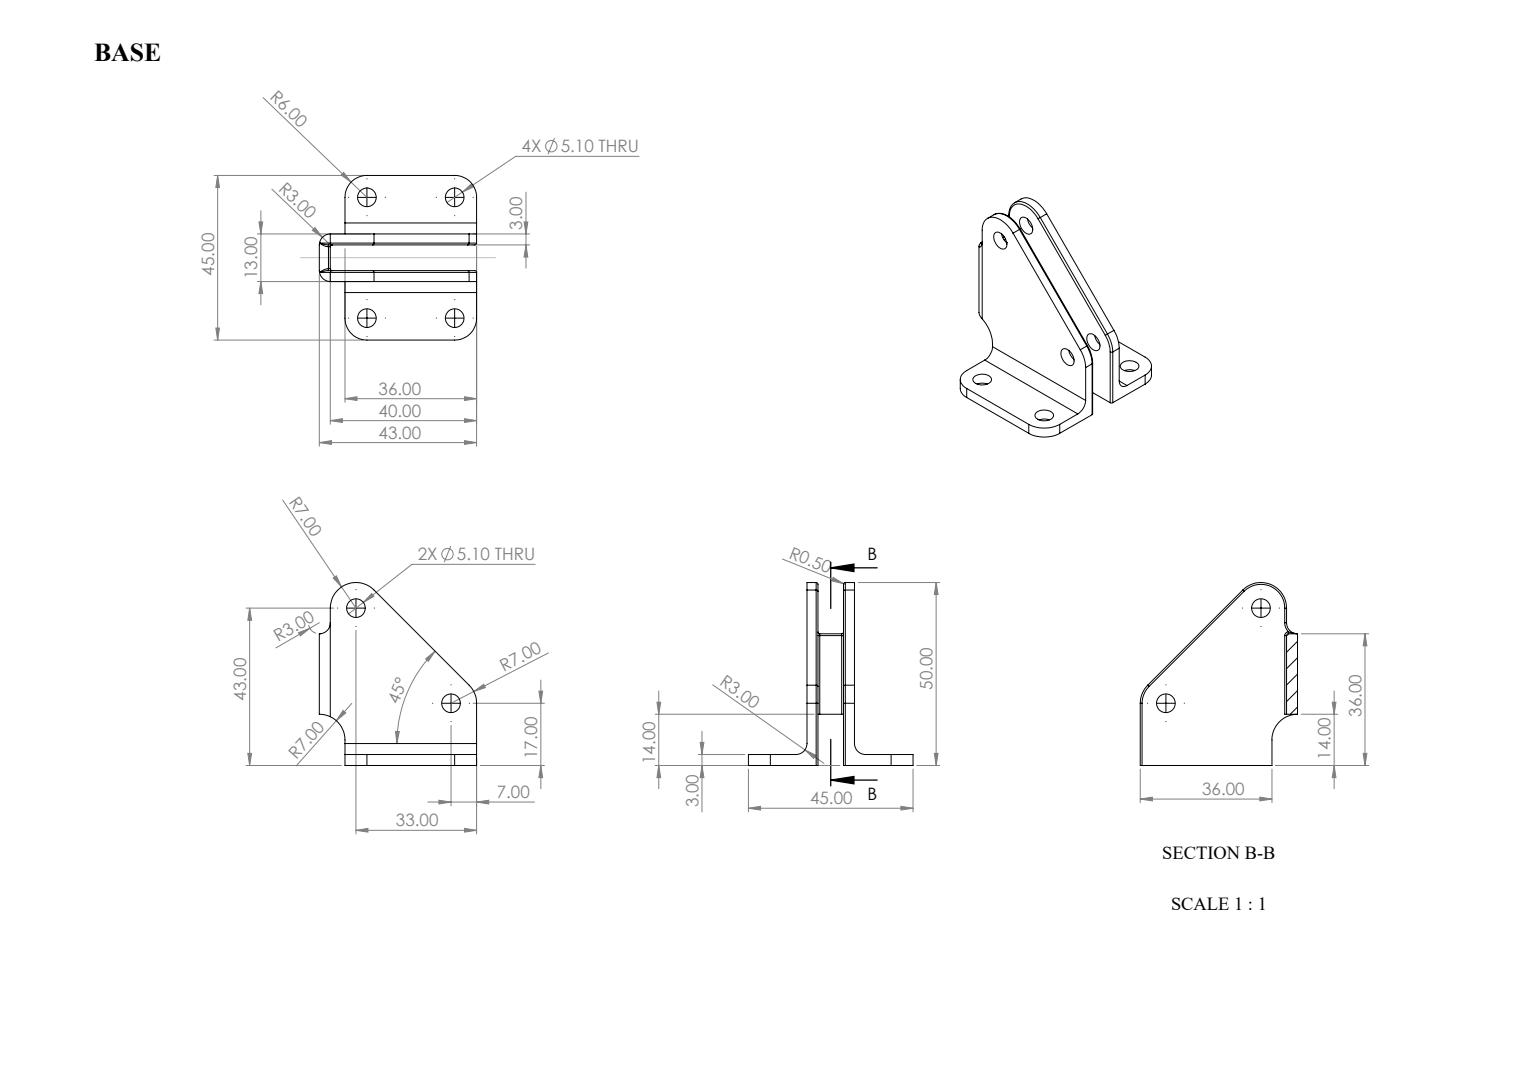
ISO-10303-21;
HEADER;
FILE_DESCRIPTION (('STEP AP214'),
    '1' );
FILE_NAME ('Base.step',
    '2026-10-06T08:09:25',
    ( '' ),
    ( '' ),
    'SwSTEP 2.0',
    'SolidWorks 2021',
    '' );
FILE_SCHEMA (( 'AUTOMOTIVE_DESIGN' ));
ENDSEC;

DATA;
#2=DIRECTION ( 'NONE',  ( -0.000000000000000000, 1.000000000000000000, -0.000000000000000000 ) ) ;
#5=CARTESIAN_POINT ( 'NONE',  ( -4.711587335153455847, 35.99999999900384751, -25.94668155291150313 ) ) ;
#7=AXIS2_PLACEMENT_3D ( 'NONE', #12336, #20843, #10124 ) ;
#19=EDGE_CURVE ( 'NONE', #13411, #2264, #4371, .T. ) ;
#28=ORIENTED_EDGE ( 'NONE', *, *, #13424, .F. ) ;
#32=EDGE_CURVE ( 'NONE', #19371, #4871, #12562, .T. ) ;
#40=CIRCLE ( 'NONE', #19182, 2.550000000000002043 ) ;
#65=ORIENTED_EDGE ( 'NONE', *, *, #2173, .F. ) ;
#84=VERTEX_POINT ( 'NONE', #16838 ) ;
#124=LINE ( 'NONE', #8704, #11013 ) ;
#134=DIRECTION ( 'NONE',  ( 1.000000000000000000, 0.000000000000000000, 0.000000000000000000 ) ) ;
#135=CIRCLE ( 'NONE', #13271, 0.5000000000000004441 ) ;
#145=VERTEX_POINT ( 'NONE', #20516 ) ;
#146=ORIENTED_EDGE ( 'NONE', *, *, #6538, .T. ) ;
#151=AXIS2_PLACEMENT_3D ( 'NONE', #11597, #19127, #20797 ) ;
#166=DIRECTION ( 'NONE',  ( -0.7071067811865475727, -0.7071067811865475727, 0.000000000000000000 ) ) ;
#176=EDGE_LOOP ( 'NONE', ( #1008, #14393, #11718, #4703 ) ) ;
#178=VERTEX_POINT ( 'NONE', #19086 ) ;
#191=STYLED_ITEM ( 'NONE', ( #6397 ), #12837 ) ;
#194=LINE ( 'NONE', #770, #19044 ) ;
#199=ORIENTED_EDGE ( 'NONE', *, *, #4642, .F. ) ;
#204=EDGE_CURVE ( 'NONE', #21236, #14256, #17064, .T. ) ;
#206=FACE_OUTER_BOUND ( 'NONE', #13645, .T. ) ;
#249=VECTOR ( 'NONE', #5863, 1000.000000000000000 ) ;
#250=ORIENTED_EDGE ( 'NONE', *, *, #16395, .F. ) ;
#251=ORIENTED_EDGE ( 'NONE', *, *, #16111, .T. ) ;
#256=DIRECTION ( 'NONE',  ( 0.000000000000000000, -1.000000000000000000, 0.000000000000000000 ) ) ;
#260=CARTESIAN_POINT ( 'NONE',  ( 6.000000000291855429, -0.5000000009961480529, -5.999999999999998224 ) ) ;
#261=DIRECTION ( 'NONE',  ( 0.000000000000000000, 0.000000000000000000, -1.000000000000000000 ) ) ;
#263=LINE ( 'NONE', #5220, #12168 ) ;
#283=VERTEX_POINT ( 'NONE', #1674 ) ;
#297=ADVANCED_FACE ( 'NONE', ( #7100 ), #21448, .T. ) ;
#301=AXIS2_PLACEMENT_3D ( 'NONE', #1691, #21234, #5101 ) ;
#325=EDGE_CURVE ( 'NONE', #4761, #2725, #5554, .T. ) ;
#327=VECTOR ( 'NONE', #12053, 1000.000000000000000 ) ;
#328=CARTESIAN_POINT ( 'NONE',  ( 2.918498775983380256E-10, 2.999999999003851503, -39.00000000000000000 ) ) ;
#334=PLANE ( 'NONE',  #18718 ) ;
#340=CARTESIAN_POINT ( 'NONE',  ( -4.614318463248865854, 37.16513102274245028, -28.94121189041531750 ) ) ;
#343=VERTEX_POINT ( 'NONE', #19786 ) ;
#344=AXIS2_PLACEMENT_3D ( 'NONE', #676, #7844, #18658 ) ;
#348=EDGE_CURVE ( 'NONE', #1547, #16744, #12832, .T. ) ;
#356=CARTESIAN_POINT ( 'NONE',  ( 26.45000000029184051, 16.99999999900385461, -19.00000000000000355 ) ) ;
#371=VERTEX_POINT ( 'NONE', #2699 ) ;
#376=CARTESIAN_POINT ( 'NONE',  ( -3.999999999708139686, 49.99999999900385461, -29.00000000000000355 ) ) ;
#379=DIRECTION ( 'NONE',  ( -0.000000000000000000, -0.000000000000000000, 1.000000000000000000 ) ) ;
#382=CARTESIAN_POINT ( 'NONE',  ( -4.470458892752995794, 37.36863211987452615, -16.03483522404608408 ) ) ;
#383=CYLINDRICAL_SURFACE ( 'NONE', #5439, 2.550000000000000711 ) ;
#412=DIRECTION ( 'NONE',  ( -1.000000000000000000, 0.000000000000000000, 0.000000000000000000 ) ) ;
#414=DIRECTION ( 'NONE',  ( 1.000000000000000000, 0.000000000000000000, 0.000000000000000000 ) ) ;
#459=VECTOR ( 'NONE', #20546, 1000.000000000000000 ) ;
#464=DIRECTION ( 'NONE',  ( 0.000000000000000000, 0.000000000000000000, 1.000000000000000000 ) ) ;
#496=CIRCLE ( 'NONE', #23096, 2.999999999999999112 ) ;
#497=DIRECTION ( 'NONE',  ( -0.7071067811865475727, -0.7071067811865475727, 0.000000000000000000 ) ) ;
#499=DIRECTION ( 'NONE',  ( -1.000000000000000000, -0.000000000000000000, -0.000000000000000000 ) ) ;
#514=AXIS2_PLACEMENT_3D ( 'NONE', #18460, #4209, #9413 ) ;
#516=EDGE_LOOP ( 'NONE', ( #5719, #17219, #15403, #12098, #8144, #13153, #18199, #8414 ) ) ;
#524=EDGE_LOOP ( 'NONE', ( #13786, #13583, #662, #2799 ) ) ;
#536=LINE ( 'NONE', #21829, #14939 ) ;
#548=ORIENTED_EDGE ( 'NONE', *, *, #14303, .F. ) ;
#555=VERTEX_POINT ( 'NONE', #22710 ) ;
#561=CARTESIAN_POINT ( 'NONE',  ( -6.958637496983413051, 36.00028509578874747, -18.50353548315064600 ) ) ;
#569=DIRECTION ( 'NONE',  ( 0.000000000000000000, 0.000000000000000000, 1.000000000000000000 ) ) ;
#603=AXIS2_PLACEMENT_3D ( 'NONE', #12913, #2082, #19970 ) ;
#615=DIRECTION ( 'NONE',  ( 1.000000000000000000, 0.000000000000000000, 0.000000000000000000 ) ) ;
#622=DIRECTION ( 'NONE',  ( -0.7071067811865475727, 0.7071067811865475727, 0.000000000000000000 ) ) ;
#638=CIRCLE ( 'NONE', #21682, 2.550000000000002043 ) ;
#645=AXIS2_PLACEMENT_3D ( 'NONE', #22990, #1692, #8628 ) ;
#662=ORIENTED_EDGE ( 'NONE', *, *, #21476, .T. ) ;
#666=CARTESIAN_POINT ( 'NONE',  ( 2.918498775983380256E-10, 2.999999999003851503, -12.99999999999999822 ) ) ;
#674=AXIS2_PLACEMENT_3D ( 'NONE', #8315, #8440, #20912 ) ;
#676=CARTESIAN_POINT ( 'NONE',  ( 30.00000000029184832, -0.5000000009961480529, -5.999999999999998224 ) ) ;
#688=VERTEX_POINT ( 'NONE', #10911 ) ;
#689=ORIENTED_EDGE ( 'NONE', *, *, #18622, .F. ) ;
#690=VERTEX_POINT ( 'NONE', #12574 ) ;
#692=AXIS2_PLACEMENT_3D ( 'NONE', #16136, #3905, #12614 ) ;
#695=EDGE_LOOP ( 'NONE', ( #13875, #14287, #3852, #8721 ) ) ;
#703=CARTESIAN_POINT ( 'NONE',  ( 36.00000000029184832, 2.999999999003851503, -5.999999999999998224 ) ) ;
#729=CARTESIAN_POINT ( 'NONE',  ( -4.239424077913610311, 37.80035007138371839, -16.00730726111445534 ) ) ;
#731=DIRECTION ( 'NONE',  ( 0.000000000000000000, 0.000000000000000000, 1.000000000000000000 ) ) ;
#736=VECTOR ( 'NONE', #1530, 1000.000000000000000 ) ;
#739=CARTESIAN_POINT ( 'NONE',  ( 6.000000000291855429, -9.961476088449217059E-10, -39.00000000000000000 ) ) ;
#750=LINE ( 'NONE', #7915, #20802 ) ;
#754=DIRECTION ( 'NONE',  ( 0.000000000000000000, 0.000000000000000000, 1.000000000000000000 ) ) ;
#762=DIRECTION ( 'NONE',  ( -0.000000000000000000, 1.000000000000000000, -0.000000000000000000 ) ) ;
#770=CARTESIAN_POINT ( 'NONE',  ( 2.918498775983380256E-10, -9.961476088449217059E-10, -45.00000000000000000 ) ) ;
#775=EDGE_LOOP ( 'NONE', ( #12033, #10591 ) ) ;
#790=CYLINDRICAL_SURFACE ( 'NONE', #17982, 2.550000000000003819 ) ;
#818=DIRECTION ( 'NONE',  ( -0.000000000000000000, 1.000000000000000000, -0.000000000000000000 ) ) ;
#819=CARTESIAN_POINT ( 'NONE',  ( 2.918498775983380256E-10, 2.999999999003851503, -29.00000000000000355 ) ) ;
#820=LINE ( 'NONE', #15157, #19828 ) ;
#827=ORIENTED_EDGE ( 'NONE', *, *, #22142, .T. ) ;
#832=DIRECTION ( 'NONE',  ( -1.000000000000000000, 0.000000000000000000, 0.000000000000000000 ) ) ;
#839=DIRECTION ( 'NONE',  ( 0.7071067811865474617, -0.7071067811865474617, 0.000000000000000000 ) ) ;
#845=DIRECTION ( 'NONE',  ( 0.000000000000000000, 1.000000000000000000, 0.000000000000000000 ) ) ;
#856=AXIS2_PLACEMENT_3D ( 'NONE', #18442, #7510, #21754 ) ;
#866=EDGE_LOOP ( 'NONE', ( #15194, #20184, #2377, #21781 ) ) ;
#888=VERTEX_POINT ( 'NONE', #16668 ) ;
#889=VECTOR ( 'NONE', #18743, 1000.000000000000000 ) ;
#944=DIRECTION ( 'NONE',  ( -1.000000000000000000, -0.000000000000000000, -0.000000000000000000 ) ) ;
#946=CARTESIAN_POINT ( 'NONE',  ( -6.999999999708142795, 38.99999999900385461, -19.00000000000000355 ) ) ;
#949=ORIENTED_EDGE ( 'NONE', *, *, #8818, .F. ) ;
#974=EDGE_CURVE ( 'NONE', #18076, #3151, #3624, .T. ) ;
#983=EDGE_LOOP ( 'NONE', ( #1133, #3126, #6569, #4982 ) ) ;
#984=CARTESIAN_POINT ( 'NONE',  ( -6.999999999708142795, 13.99999999900385106, -22.50000000000000000 ) ) ;
#987=FACE_OUTER_BOUND ( 'NONE', #17816, .T. ) ;
#989=DIRECTION ( 'NONE',  ( -0.000000000000000000, -0.000000000000000000, 1.000000000000000000 ) ) ;
#993=CARTESIAN_POINT ( 'NONE',  ( 30.00000000029184832, -9.961476088449217059E-10, -39.00000000000000000 ) ) ;
#996=FACE_OUTER_BOUND ( 'NONE', #14966, .T. ) ;
#1008=ORIENTED_EDGE ( 'NONE', *, *, #19202, .T. ) ;
#1009=ORIENTED_EDGE ( 'NONE', *, *, #10614, .F. ) ;
#1010=AXIS2_PLACEMENT_3D ( 'NONE', #8199, #4301, #10078 ) ;
#1013=VECTOR ( 'NONE', #7217, 1000.000000000000000 ) ;
#1016=DIRECTION ( 'NONE',  ( 1.000000000000000000, -1.858632295689435609E-16, 0.000000000000000000 ) ) ;
#1017=DIRECTION ( 'NONE',  ( 1.000000000000000000, 0.000000000000000000, 0.000000000000000000 ) ) ;
#1018=ADVANCED_FACE ( 'NONE', ( #13625 ), #18923, .F. ) ;
#1020=CARTESIAN_POINT ( 'NONE',  ( -6.999999999708142795, 35.99999999900384751, -22.50000000000000000 ) ) ;
#1024=FACE_BOUND ( 'NONE', #9944, .T. ) ;
#1027=B_SPLINE_CURVE_WITH_KNOTS ( 'NONE', 3,
 ( #21795, #5679, #12838, #11417, #18604, #18254, #22246, #4347, #6134, #2477, #9315, #9656, #13313, #16811, #382, #729, #20493, #11527, #16358, #21901 ),
 .UNSPECIFIED., .F., .F.,
 ( 4, 2, 2, 2, 2, 2, 2, 2, 2, 4 ),
 ( 0.0005000078514897923158, 0.001232179299099195411, 0.001964350746708598289, 0.002696522194318001601, 0.003062607918122696102, 0.003428693641927389735, 0.004160865089536783072, 0.004893036537146174675, 0.005625207984755568012, 0.006357379432364960482 ),
 .UNSPECIFIED. ) ;
#1034=FACE_OUTER_BOUND ( 'NONE', #5261, .T. ) ;
#1036=AXIS2_PLACEMENT_3D ( 'NONE', #946, #10108, #20935 ) ;
#1046=FACE_OUTER_BOUND ( 'NONE', #14257, .T. ) ;
#1058=EDGE_CURVE ( 'NONE', #11848, #1430, #638, .T. ) ;
#1061=DIRECTION ( 'NONE',  ( -1.613696256722611405E-16, 0.000000000000000000, -1.000000000000000000 ) ) ;
#1066=AXIS2_PLACEMENT_3D ( 'NONE', #3230, #21463, #8745 ) ;
#1068=ADVANCED_FACE ( 'NONE', ( #1046 ), #15491, .F. ) ;
#1077=CARTESIAN_POINT ( 'NONE',  ( -6.549842551586334771, 36.00336057837468928, -26.38138186026117893 ) ) ;
#1082=CARTESIAN_POINT ( 'NONE',  ( 35.50000000029184832, 2.999999999003851503, -19.00000000000000355 ) ) ;
#1087=CARTESIAN_POINT ( 'NONE',  ( 35.50000000029184832, 2.999999999003851503, -18.50000000000000355 ) ) ;
#1090=AXIS2_PLACEMENT_3D ( 'NONE', #17003, #17354, #15598 ) ;
#1103=ORIENTED_EDGE ( 'NONE', *, *, #6153, .T. ) ;
#1127=ORIENTED_EDGE ( 'NONE', *, *, #8585, .T. ) ;
#1130=AXIS2_PLACEMENT_3D ( 'NONE', #16695, #21064, #22587 ) ;
#1133=ORIENTED_EDGE ( 'NONE', *, *, #7575, .T. ) ;
#1137=DIRECTION ( 'NONE',  ( 0.000000000000000000, -1.000000000000000000, 0.000000000000000000 ) ) ;
#1142=CARTESIAN_POINT ( 'NONE',  ( -6.962001439796708269, 35.99999999900384751, -26.47597002942762145 ) ) ;
#1153=EDGE_CURVE ( 'NONE', #19243, #10116, #19375, .T. ) ;
#1163=DIRECTION ( 'NONE',  ( 0.000000000000000000, 0.000000000000000000, 1.000000000000000000 ) ) ;
#1169=CARTESIAN_POINT ( 'NONE',  ( 2.918498775983380256E-10, 6.999999999003851947, -26.00000000000000000 ) ) ;
#1181=ORIENTED_EDGE ( 'NONE', *, *, #21353, .T. ) ;
#1234=ORIENTED_EDGE ( 'NONE', *, *, #8668, .F. ) ;
#1245=ORIENTED_EDGE ( 'NONE', *, *, #3629, .T. ) ;
#1257=VECTOR ( 'NONE', #20720, 1000.000000000000000 ) ;
#1267=ORIENTED_EDGE ( 'NONE', *, *, #2745, .T. ) ;
#1276=AXIS2_PLACEMENT_3D ( 'NONE', #16097, #15759, #12105 ) ;
#1296=TOROIDAL_SURFACE ( 'NONE', #11415, 6.500000000000000888, 0.5000000000000000000 ) ;
#1305=ORIENTED_EDGE ( 'NONE', *, *, #10538, .T. ) ;
#1325=VECTOR ( 'NONE', #1887, 1000.000000000000000 ) ;
#1354=ORIENTED_EDGE ( 'NONE', *, *, #16873, .F. ) ;
#1364=DIRECTION ( 'NONE',  ( 1.000000000000000000, 0.000000000000000000, 0.000000000000000000 ) ) ;
#1370=CARTESIAN_POINT ( 'NONE',  ( -6.959227686631209941, 36.00023952070644384, -18.50706566189541391 ) ) ;
#1376=CARTESIAN_POINT ( 'NONE',  ( -5.786576545576803454, 13.89610628501159795, -16.58192921595065883 ) ) ;
#1412=AXIS2_PLACEMENT_3D ( 'NONE', #8513, #19100, #13917 ) ;
#1413=ORIENTED_EDGE ( 'NONE', *, *, #10933, .T. ) ;
#1425=APPLICATION_CONTEXT ( 'automotive_design' ) ;
#1430=VERTEX_POINT ( 'NONE', #15434 ) ;
#1432=ADVANCED_FACE ( 'NONE', ( #22976 ), #12015, .F. ) ;
#1451=DIRECTION ( 'NONE',  ( 0.000000000000000000, 1.000000000000000000, -0.000000000000000000 ) ) ;
#1500=CARTESIAN_POINT ( 'NONE',  ( 29.00000000029184832, 16.99999999900385461, -25.50000000000000355 ) ) ;
#1510=DIRECTION ( 'NONE',  ( 1.000000000000000000, -0.000000000000000000, -0.000000000000000000 ) ) ;
#1520=VERTEX_POINT ( 'NONE', #10375 ) ;
#1530=DIRECTION ( 'NONE',  ( -1.000000000000000000, 0.000000000000000000, -0.000000000000000000 ) ) ;
#1534=DIRECTION ( 'NONE',  ( -1.000000000000000000, 0.000000000000000000, 0.000000000000000000 ) ) ;
#1537=AXIS2_PLACEMENT_3D ( 'NONE', #19881, #3750, #9051 ) ;
#1541=EDGE_LOOP ( 'NONE', ( #19704, #15907, #14735, #4989 ) ) ;
#1544=ORIENTED_EDGE ( 'NONE', *, *, #20662, .F. ) ;
#1547=VERTEX_POINT ( 'NONE', #5448 ) ;
#1577=CARTESIAN_POINT ( 'NONE',  ( 2.918498775983380256E-10, -9.961476088449217059E-10, -26.00000000000000000 ) ) ;
#1597=EDGE_CURVE ( 'NONE', #20279, #8964, #13375, .T. ) ;
#1602=ORIENTED_EDGE ( 'NONE', *, *, #4180, .F. ) ;
#1628=EDGE_CURVE ( 'NONE', #14201, #16629, #12993, .T. ) ;
#1648=EDGE_CURVE ( 'NONE', #15365, #9160, #13753, .T. ) ;
#1655=VECTOR ( 'NONE', #17115, 1000.000000000000000 ) ;
#1665=VERTEX_POINT ( 'NONE', #15051 ) ;
#1670=AXIS2_PLACEMENT_3D ( 'NONE', #6502, #15199, #22268 ) ;
#1674=CARTESIAN_POINT ( 'NONE',  ( -3.999999999708153453, 38.99999999900385461, -15.99999999999999289 ) ) ;
#1681=EDGE_CURVE ( 'NONE', #8658, #12443, #16806, .T. ) ;
#1683=FACE_OUTER_BOUND ( 'NONE', #1741, .T. ) ;
#1688=LINE ( 'NONE', #5330, #1013 ) ;
#1691=CARTESIAN_POINT ( 'NONE',  ( -4.499999999708154341, 35.49999999900384751, -25.50000000000000000 ) ) ;
#1692=DIRECTION ( 'NONE',  ( 0.000000000000000000, 0.000000000000000000, 1.000000000000000000 ) ) ;
#1703=DIRECTION ( 'NONE',  ( -1.858632295689435609E-16, -1.000000000000000000, 0.000000000000000000 ) ) ;
#1710=PLANE ( 'NONE',  #19487 ) ;
#1720=ORIENTED_EDGE ( 'NONE', *, *, #15193, .T. ) ;
#1722=ORIENTED_EDGE ( 'NONE', *, *, #14532, .T. ) ;
#1741=EDGE_LOOP ( 'NONE', ( #12035, #6194, #22439, #10055 ) ) ;
#1747=AXIS2_PLACEMENT_3D ( 'NONE', #8327, #15376, #7978 ) ;
#1765=CARTESIAN_POINT ( 'NONE',  ( -4.499999999708154341, 35.99999999900384751, -22.50000000000000000 ) ) ;
#1780=CARTESIAN_POINT ( 'NONE',  ( -6.962001439796708269, 35.99999999900384751, -26.47597002942762145 ) ) ;
#1782=CARTESIAN_POINT ( 'NONE',  ( 29.00000000029184832, 16.99999999900385461, -18.50000000000000355 ) ) ;
#1787=EDGE_CURVE ( 'NONE', #9785, #9160, #6352, .T. ) ;
#1802=ORIENTED_EDGE ( 'NONE', *, *, #17536, .F. ) ;
#1811=ORIENTED_EDGE ( 'NONE', *, *, #2933, .F. ) ;
#1820=DIRECTION ( 'NONE',  ( 0.000000000000000000, 0.000000000000000000, 1.000000000000000000 ) ) ;
#1824=CARTESIAN_POINT ( 'NONE',  ( -4.365918574175959854, 13.48846683486500808, -16.01652206364978781 ) ) ;
#1833=ORIENTED_EDGE ( 'NONE', *, *, #348, .F. ) ;
#1834=VERTEX_POINT ( 'NONE', #19062 ) ;
#1842=DIRECTION ( 'NONE',  ( 0.000000000000000000, -0.000000000000000000, -1.000000000000000000 ) ) ;
#1845=LINE ( 'NONE', #5152, #3945 ) ;
#1857=ORIENTED_EDGE ( 'NONE', *, *, #6505, .F. ) ;
#1858=CARTESIAN_POINT ( 'NONE',  ( -6.226186441994419063, 36.09747688189035131, -28.02588720118439269 ) ) ;
#1887=DIRECTION ( 'NONE',  ( 0.000000000000000000, -1.000000000000000000, 0.000000000000000000 ) ) ;
#1891=CARTESIAN_POINT ( 'NONE',  ( 0.4500000002918510544, 42.99999999900385461, -15.99999999999999289 ) ) ;
#1911=ORIENTED_EDGE ( 'NONE', *, *, #17784, .T. ) ;
#1914=ORIENTED_EDGE ( 'NONE', *, *, #5831, .T. ) ;
#1915=ORIENTED_EDGE ( 'NONE', *, *, #4798, .F. ) ;
#1916=EDGE_LOOP ( 'NONE', ( #16349, #12628 ) ) ;
#1933=CARTESIAN_POINT ( 'NONE',  ( 5.550000000291854363, 42.99999999900385461, -25.50000000000000355 ) ) ;
#1952=FACE_BOUND ( 'NONE', #15450, .T. ) ;
#1954=CARTESIAN_POINT ( 'NONE',  ( 2.918498775983380256E-10, -9.961476088449217059E-10, -19.00000000000000355 ) ) ;
#1974=CARTESIAN_POINT ( 'NONE',  ( -6.959810536856695151, 36.00015702695179698, -18.51059057611807646 ) ) ;
#1993=CIRCLE ( 'NONE', #20796, 0.5000000000000004441 ) ;
#2011=CIRCLE ( 'NONE', #9164, 2.550000000000002043 ) ;
#2025=CARTESIAN_POINT ( 'NONE',  ( -5.416517661024267127, 35.99999999900385461, -19.34908248715211698 ) ) ;
#2035=ORIENTED_EDGE ( 'NONE', *, *, #21054, .T. ) ;
#2041=ORIENTED_EDGE ( 'NONE', *, *, #13149, .F. ) ;
#2049=LINE ( 'NONE', #18181, #15713 ) ;
#2054=FACE_OUTER_BOUND ( 'NONE', #6213, .T. ) ;
#2057=CYLINDRICAL_SURFACE ( 'NONE', #5233, 3.000000000000002665 ) ;
#2058=ORIENTED_EDGE ( 'NONE', *, *, #21821, .T. ) ;
#2068=DIRECTION ( 'NONE',  ( -0.000000000000000000, -0.000000000000000000, 1.000000000000000000 ) ) ;
#2075=CARTESIAN_POINT ( 'NONE',  ( 6.000000000291855429, -9.961476088449217059E-10, -5.999999999999998224 ) ) ;
#2076=DIRECTION ( 'NONE',  ( 0.000000000000000000, 0.000000000000000000, -1.000000000000000000 ) ) ;
#2079=CARTESIAN_POINT ( 'NONE',  ( -3.999999999708153453, 13.99999999900385106, -25.50000000000000000 ) ) ;
#2082=DIRECTION ( 'NONE',  ( 0.000000000000000000, 0.000000000000000000, 1.000000000000000000 ) ) ;
#2085=ORIENTED_EDGE ( 'NONE', *, *, #12867, .F. ) ;
#2087=CARTESIAN_POINT ( 'NONE',  ( -5.688936712956119024, 36.29949271875472050, -28.48196112119369872 ) ) ;
#2098=AXIS2_PLACEMENT_3D ( 'NONE', #16122, #18136, #7434 ) ;
#2114=AXIS2_PLACEMENT_3D ( 'NONE', #21381, #3259, #10764 ) ;
#2120=CARTESIAN_POINT ( 'NONE',  ( 6.000000000291855429, -0.5000000009961480529, -36.44999999999999574 ) ) ;
#2131=DIRECTION ( 'NONE',  ( 0.000000000000000000, 0.000000000000000000, 1.000000000000000000 ) ) ;
#2132=CIRCLE ( 'NONE', #645, 7.000000000000006217 ) ;
#2136=AXIS2_PLACEMENT_3D ( 'NONE', #16578, #13075, #18712 ) ;
#2149=ORIENTED_EDGE ( 'NONE', *, *, #14274, .F. ) ;
#2151=AXIS2_PLACEMENT_3D ( 'NONE', #13612, #17479, #13377 ) ;
#2153=ORIENTED_EDGE ( 'NONE', *, *, #17447, .F. ) ;
#2161=CIRCLE ( 'NONE', #9694, 0.5000000000000004441 ) ;
#2164=CYLINDRICAL_SURFACE ( 'NONE', #12544, 6.000000000000000000 ) ;
#2173=EDGE_CURVE ( 'NONE', #1520, #13097, #19438, .T. ) ;
#2189=STYLED_ITEM ( 'NONE', ( #15993 ), #18435 ) ;
#2192=DIRECTION ( 'NONE',  ( 0.000000000000000000, -1.000000000000000000, 0.000000000000000000 ) ) ;
#2195=EDGE_CURVE ( 'NONE', #22557, #6752, #7982, .T. ) ;
#2216=AXIS2_PLACEMENT_3D ( 'NONE', #8310, #9965, #4539 ) ;
#2222=CARTESIAN_POINT ( 'NONE',  ( 3.000000000291852764, 42.99999999900385461, -29.00000000000000355 ) ) ;
#2229=DIRECTION ( 'NONE',  ( -0.000000000000000000, 1.000000000000000000, -0.000000000000000000 ) ) ;
#2236=PRODUCT_CONTEXT ( 'NONE', #4265, 'mechanical' ) ;
#2241=ORIENTED_EDGE ( 'NONE', *, *, #19442, .F. ) ;
#2244=B_SPLINE_CURVE_WITH_KNOTS ( 'NONE', 3,
 ( #6710, #1077, #3060, #4928, #12096, #17395, #20947, #6949 ),
 .UNSPECIFIED., .F., .F.,
 ( 4, 2, 2, 4 ),
 ( 1.379105163401561640E-16, 0.001256837924491785441, 0.001885256886737605954, 0.002513675848983426466 ),
 .UNSPECIFIED. ) ;
#2249=DIRECTION ( 'NONE',  ( 0.000000000000000000, -1.000000000000000000, 0.000000000000000000 ) ) ;
#2255=CARTESIAN_POINT ( 'NONE',  ( 29.00000000029184832, 16.99999999900385461, -29.00000000000000355 ) ) ;
#2258=LINE ( 'NONE', #18611, #10431 ) ;
#2264=VERTEX_POINT ( 'NONE', #6577 ) ;
#2284=DIRECTION ( 'NONE',  ( 0.000000000000000000, 0.000000000000000000, -1.000000000000000000 ) ) ;
#2286=CARTESIAN_POINT ( 'NONE',  ( 30.00000000029184832, -9.961476088449217059E-10, -8.549999999999997158 ) ) ;
#2288=DIRECTION ( 'NONE',  ( 1.000000000000000000, 0.000000000000000000, 0.000000000000000000 ) ) ;
#2292=VERTEX_POINT ( 'NONE', #11966 ) ;
#2294=VERTEX_POINT ( 'NONE', #10100 ) ;
#2300=ORIENTED_EDGE ( 'NONE', *, *, #23059, .F. ) ;
#2313=EDGE_CURVE ( 'NONE', #22269, #6361, #17197, .T. ) ;
#2319=VERTEX_POINT ( 'NONE', #10674 ) ;
#2338=DIRECTION ( 'NONE',  ( -0.000000000000000000, -0.000000000000000000, 1.000000000000000000 ) ) ;
#2353=ORIENTED_EDGE ( 'NONE', *, *, #12867, .T. ) ;
#2356=DIRECTION ( 'NONE',  ( -1.858632295689435609E-16, -1.000000000000000000, 0.000000000000000000 ) ) ;
#2358=DIRECTION ( 'NONE',  ( 0.000000000000000000, 0.000000000000000000, 1.000000000000000000 ) ) ;
#2377=ORIENTED_EDGE ( 'NONE', *, *, #9962, .T. ) ;
#2378=ORIENTED_EDGE ( 'NONE', *, *, #15996, .T. ) ;
#2379=ORIENTED_EDGE ( 'NONE', *, *, #7246, .T. ) ;
#2384=AXIS2_PLACEMENT_3D ( 'NONE', #20464, #818, #15260 ) ;
#2388=DIRECTION ( 'NONE',  ( 0.000000000000000000, 0.000000000000000000, -1.000000000000000000 ) ) ;
#2392=ORIENTED_EDGE ( 'NONE', *, *, #9910, .F. ) ;
#2400=DIRECTION ( 'NONE',  ( 1.858632295689435609E-16, 1.000000000000000000, 0.000000000000000000 ) ) ;
#2428=CARTESIAN_POINT ( 'NONE',  ( 36.00000000029184832, -9.961476088449217059E-10, -26.50000000000000000 ) ) ;
#2431=LINE ( 'NONE', #5744, #249 ) ;
#2454=DIRECTION ( 'NONE',  ( -0.000000000000000000, -0.000000000000000000, 1.000000000000000000 ) ) ;
#2461=CIRCLE ( 'NONE', #7000, 3.000000000000002665 ) ;
#2466=ADVANCED_FACE ( 'NONE', ( #12550, #12192, #3618 ), #10784, .T. ) ;
#2467=ORIENTED_EDGE ( 'NONE', *, *, #18247, .T. ) ;
#2477=CARTESIAN_POINT ( 'NONE',  ( -5.498446330623520062, 36.40058408549440117, -16.39859714349349673 ) ) ;
#2544=LINE ( 'NONE', #9732, #1655 ) ;
#2550=CARTESIAN_POINT ( 'NONE',  ( 33.59619407800441593, 21.59619407671642222, -26.00000000000000000 ) ) ;
#2568=CIRCLE ( 'NONE', #7466, 2.999999999999999112 ) ;
#2608=EDGE_CURVE ( 'NONE', #3717, #14311, #20313, .T. ) ;
#2611=ORIENTED_EDGE ( 'NONE', *, *, #1787, .F. ) ;
#2623=EDGE_CURVE ( 'NONE', #3689, #12152, #5622, .T. ) ;
#2624=SURFACE_STYLE_USAGE ( .BOTH. , #18851 ) ;
#2632=DIRECTION ( 'NONE',  ( -1.000000000000000000, 0.000000000000000000, 1.613696256722611405E-16 ) ) ;
#2647=ORIENTED_EDGE ( 'NONE', *, *, #17863, .T. ) ;
#2651=DIRECTION ( 'NONE',  ( -1.000000000000000000, -0.000000000000000000, 1.613696256722611405E-16 ) ) ;
#2664=CARTESIAN_POINT ( 'NONE',  ( 6.000000000291855429, 2.999999999003851503, 0.000000000000000000 ) ) ;
#2675=EDGE_LOOP ( 'NONE', ( #8873, #5208, #5490, #18056 ) ) ;
#2679=CARTESIAN_POINT ( 'NONE',  ( -6.975867733769219647, 36.00005661733510465, -18.50635935043928981 ) ) ;
#2685=CARTESIAN_POINT ( 'NONE',  ( 30.00000000029184832, 2.999999999003851503, -5.999999999999998224 ) ) ;
#2687=AXIS2_PLACEMENT_3D ( 'NONE', #8853, #14682, #16009 ) ;
#2691=ADVANCED_FACE ( 'NONE', ( #17109 ), #790, .F. ) ;
#2698=DIRECTION ( 'NONE',  ( 0.000000000000000000, 0.000000000000000000, -1.000000000000000000 ) ) ;
#2699=CARTESIAN_POINT ( 'NONE',  ( 30.00000000029184832, 2.999999999003851503, -3.449999999999999289 ) ) ;
#2713=CIRCLE ( 'NONE', #17752, 2.999999999999999112 ) ;
#2725=VERTEX_POINT ( 'NONE', #15586 ) ;
#2732=ADVANCED_FACE ( 'NONE', ( #19014 ), #13487, .F. ) ;
#2745=EDGE_CURVE ( 'NONE', #2319, #5235, #5570, .T. ) ;
#2749=CARTESIAN_POINT ( 'NONE',  ( 6.000000000291855429, -9.961476088449217059E-10, -8.549999999999998934 ) ) ;
#2756=EDGE_LOOP ( 'NONE', ( #17452, #7889, #14961, #19393 ) ) ;
#2760=AXIS2_PLACEMENT_3D ( 'NONE', #16922, #2698, #8347 ) ;
#2767=CARTESIAN_POINT ( 'NONE',  ( 7.949747468597695210, 47.94974746730969173, -15.99999999999999289 ) ) ;
#2771=ORIENTED_EDGE ( 'NONE', *, *, #17419, .F. ) ;
#2773=EDGE_CURVE ( 'NONE', #11457, #2292, #3041, .T. ) ;
#2788=EDGE_CURVE ( 'NONE', #2802, #13206, #16846, .T. ) ;
#2799=ORIENTED_EDGE ( 'NONE', *, *, #9962, .F. ) ;
#2802=VERTEX_POINT ( 'NONE', #14180 ) ;
#2810=DIRECTION ( 'NONE',  ( -0.7071067811865457964, 0.7071067811865492381, 0.000000000000000000 ) ) ;
#2828=CARTESIAN_POINT ( 'NONE',  ( 33.94974746859769255, 21.94974746730969528, -26.50000000000000000 ) ) ;
#2839=CARTESIAN_POINT ( 'NONE',  ( 3.000000000291852764, 42.99999999900385461, -26.00000000000000000 ) ) ;
#2852=ORIENTED_EDGE ( 'NONE', *, *, #15065, .T. ) ;
#2854=CARTESIAN_POINT ( 'NONE',  ( -6.959810536856695151, 36.00015702695179698, -18.51059057611807646 ) ) ;
#2865=DIRECTION ( 'NONE',  ( 1.000000000000000000, 0.000000000000000000, 0.000000000000000000 ) ) ;
#2872=ORIENTED_EDGE ( 'NONE', *, *, #13029, .F. ) ;
#2887=EDGE_CURVE ( 'NONE', #5722, #22384, #2568, .T. ) ;
#2888=DIRECTION ( 'NONE',  ( -1.613696256722611405E-16, 0.000000000000000000, 1.000000000000000000 ) ) ;
#2898=ORIENTED_EDGE ( 'NONE', *, *, #21021, .F. ) ;
#2919=ADVANCED_FACE ( 'NONE', ( #10641 ), #1710, .F. ) ;
#2927=LINE ( 'NONE', #10450, #21716 ) ;
#2930=EDGE_CURVE ( 'NONE', #3151, #13641, #2049, .T. ) ;
#2932=CIRCLE ( 'NONE', #16791, 0.5000000000000004441 ) ;
#2933=EDGE_CURVE ( 'NONE', #22474, #3643, #9233, .T. ) ;
#2938=CIRCLE ( 'NONE', #5560, 2.549999999999998490 ) ;
#2940=ORIENTED_EDGE ( 'NONE', *, *, #10960, .F. ) ;
#2963=DIRECTION ( 'NONE',  ( 0.000000000000000000, 0.000000000000000000, 1.000000000000000000 ) ) ;
#2973=ORIENTED_EDGE ( 'NONE', *, *, #1153, .T. ) ;
#2974=CARTESIAN_POINT ( 'NONE',  ( 29.00000000029184832, 16.99999999900385461, -25.50000000000000355 ) ) ;
#2991=CARTESIAN_POINT ( 'NONE',  ( -6.839530184912446131, 13.99859551563898563, -26.98838964695894660 ) ) ;
#3003=ADVANCED_FACE ( 'NONE', ( #12759 ), #16461, .T. ) ;
#3010=DIRECTION ( 'NONE',  ( 1.000000000000000000, 0.000000000000000000, 0.000000000000000000 ) ) ;
#3018=DIRECTION ( 'NONE',  ( -0.7071067811865474617, 0.7071067811865474617, -0.000000000000000000 ) ) ;
#3021=LINE ( 'NONE', #4544, #13855 ) ;
#3026=ORIENTED_EDGE ( 'NONE', *, *, #15093, .T. ) ;
#3041=B_SPLINE_CURVE_WITH_KNOTS ( 'NONE', 3,
 ( #19714, #22894, #8886, #10528 ),
 .UNSPECIFIED., .F., .F.,
 ( 4, 4 ),
 ( 0.0007727519425873948704, 0.0007833511101368439283 ),
 .UNSPECIFIED. ) ;
#3060=CARTESIAN_POINT ( 'NONE',  ( -6.147973203409641485, 36.05667699661070458, -26.27430804596576408 ) ) ;
#3068=CARTESIAN_POINT ( 'NONE',  ( -4.499999999708154341, 35.49999999900384751, -25.50000000000000000 ) ) ;
#3074=CARTESIAN_POINT ( 'NONE',  ( 3.000000000291852764, 42.99999999900385461, -26.00000000000000000 ) ) ;
#3083=VERTEX_POINT ( 'NONE', #17082 ) ;
#3094=ADVANCED_FACE ( 'NONE', ( #7188 ), #19649, .T. ) ;
#3114=EDGE_LOOP ( 'NONE', ( #5783, #20157, #17268, #1245 ) ) ;
#3126=ORIENTED_EDGE ( 'NONE', *, *, #13856, .T. ) ;
#3140=DIRECTION ( 'NONE',  ( 0.000000000000000000, 0.000000000000000000, -1.000000000000000000 ) ) ;
#3151=VERTEX_POINT ( 'NONE', #9292 ) ;
#3169=DIRECTION ( 'NONE',  ( -1.000000000000000000, 0.000000000000000000, 0.000000000000000000 ) ) ;
#3175=ORIENTED_EDGE ( 'NONE', *, *, #12553, .F. ) ;
#3181=ORIENTED_EDGE ( 'NONE', *, *, #15093, .F. ) ;
#3193=MECHANICAL_DESIGN_GEOMETRIC_PRESENTATION_REPRESENTATION('',(#191),#16682);
#3215=DIRECTION ( 'NONE',  ( 0.000000000000000000, 0.000000000000000000, 1.000000000000000000 ) ) ;
#3220=CARTESIAN_POINT ( 'NONE',  ( 36.00000000029184832, 5.999999999003851059, -28.99999999999999645 ) ) ;
#3230=CARTESIAN_POINT ( 'NONE',  ( 29.00000000029184832, 16.99999999900385461, -19.00000000000000355 ) ) ;
#3231=EDGE_CURVE ( 'NONE', #22993, #18159, #12287, .T. ) ;
#3236=B_SPLINE_CURVE_WITH_KNOTS ( 'NONE', 3,
 ( #16776, #9398, #9278, #18224, #21984, #5641, #18102, #1974 ),
 .UNSPECIFIED., .F., .F.,
 ( 4, 2, 2, 4 ),
 ( 0.000000000000000000, 0.0006328062630452634943, 0.001265612526090526989, 0.002531225052181053543 ),
 .UNSPECIFIED. ) ;
#3243=CARTESIAN_POINT ( 'NONE',  ( 3.000000000291852764, 42.99999999900385461, -19.49999999999998934 ) ) ;
#3253=DIRECTION ( 'NONE',  ( -0.000000000000000000, 0.000000000000000000, 1.000000000000000000 ) ) ;
#3258=EDGE_CURVE ( 'NONE', #12387, #22557, #8172, .T. ) ;
#3259=DIRECTION ( 'NONE',  ( -0.000000000000000000, -0.000000000000000000, 1.000000000000000000 ) ) ;
#3276=DIRECTION ( 'NONE',  ( 0.000000000000000000, 0.000000000000000000, 1.000000000000000000 ) ) ;
#3281=CYLINDRICAL_SURFACE ( 'NONE', #5471, 2.549999999999998934 ) ;
#3283=CIRCLE ( 'NONE', #4379, 2.549999999999996714 ) ;
#3290=ORIENTED_EDGE ( 'NONE', *, *, #4682, .F. ) ;
#3310=DIRECTION ( 'NONE',  ( 0.000000000000000000, 0.000000000000000000, 1.000000000000000000 ) ) ;
#3313=DIRECTION ( 'NONE',  ( 1.000000000000000000, 0.000000000000000000, 0.000000000000000000 ) ) ;
#3317=SURFACE_STYLE_USAGE ( .BOTH. , #14128 ) ;
#3326=CARTESIAN_POINT ( 'NONE',  ( -5.416517661024182750, 35.99999999900385461, -25.65091751284785815 ) ) ;
#3340=CIRCLE ( 'NONE', #16445, 0.4999999999999994449 ) ;
#3382=CARTESIAN_POINT ( 'NONE',  ( -4.182466315668081691, 13.41110669254460852, -29.00000000000000000 ) ) ;
#3386=EDGE_CURVE ( 'NONE', #3717, #5983, #820, .T. ) ;
#3421=EDGE_CURVE ( 'NONE', #19136, #15368, #22699, .T. ) ;
#3429=ORIENTED_EDGE ( 'NONE', *, *, #9910, .T. ) ;
#3430=ORIENTED_EDGE ( 'NONE', *, *, #19341, .F. ) ;
#3437=CARTESIAN_POINT ( 'NONE',  ( -6.590924991937371580, 35.99999999900385461, -26.24135183128864313 ) ) ;
#3438=CARTESIAN_POINT ( 'NONE',  ( -3.499999999708153453, 13.99999999900385106, -26.00000000000000000 ) ) ;
#3459=EDGE_CURVE ( 'NONE', #12296, #371, #4561, .T. ) ;
#3462=ORIENTED_EDGE ( 'NONE', *, *, #5486, .F. ) ;
#3465=CARTESIAN_POINT ( 'NONE',  ( 29.00000000029184832, 16.99999999900385461, -19.49999999999998934 ) ) ;
#3470=CARTESIAN_POINT ( 'NONE',  ( 26.09619407800442659, 29.09619407671642222, -18.50000000000000355 ) ) ;
#3472=CARTESIAN_POINT ( 'NONE',  ( -3.999999999708139686, 35.99999999900384751, -26.00000000000000711 ) ) ;
#3475=EDGE_CURVE ( 'NONE', #3554, #14655, #4393, .T. ) ;
#3478=DIRECTION ( 'NONE',  ( 0.000000000000000000, 1.000000000000000000, 0.000000000000000000 ) ) ;
#3494=EDGE_CURVE ( 'NONE', #2294, #19191, #2927, .T. ) ;
#3500=AXIS2_PLACEMENT_3D ( 'NONE', #4714, #11883, #19065 ) ;
#3520=VERTEX_POINT ( 'NONE', #8570 ) ;
#3525=CARTESIAN_POINT ( 'NONE',  ( -5.523909222203892355, 35.99999999900385461, -25.97380687558948864 ) ) ;
#3538=DIRECTION ( 'NONE',  ( -0.000000000000000000, -1.000000000000000000, 0.000000000000000000 ) ) ;
#3554=VERTEX_POINT ( 'NONE', #16313 ) ;
#3559=DIRECTION ( 'NONE',  ( 1.734723475976805517E-15, 0.000000000000000000, 1.000000000000000000 ) ) ;
#3562=CARTESIAN_POINT ( 'NONE',  ( 30.00000000029184832, -9.961476088449217059E-10, 0.000000000000000000 ) ) ;
#3569=DIRECTION ( 'NONE',  ( -0.000000000000000000, -0.000000000000000000, 1.000000000000000000 ) ) ;
#3600=ORIENTED_EDGE ( 'NONE', *, *, #17872, .F. ) ;
#3606=AXIS2_PLACEMENT_3D ( 'NONE', #14709, #11412, #2358 ) ;
#3611=DIRECTION ( 'NONE',  ( 1.000000000000000000, 0.000000000000000000, 0.000000000000000000 ) ) ;
#3618=FACE_OUTER_BOUND ( 'NONE', #4252, .T. ) ;
#3620=FACE_OUTER_BOUND ( 'NONE', #15096, .T. ) ;
#3621=CARTESIAN_POINT ( 'NONE',  ( 2.918498775983380256E-10, 2.999999999003851503, 0.000000000000000000 ) ) ;
#3624=CIRCLE ( 'NONE', #16748, 2.549999999999996714 ) ;
#3629=EDGE_CURVE ( 'NONE', #12443, #7223, #21634, .T. ) ;
#3636=ADVANCED_FACE ( 'NONE', ( #8685 ), #14217, .F. ) ;
#3643=VERTEX_POINT ( 'NONE', #1954 ) ;
#3651=EDGE_CURVE ( 'NONE', #19572, #18888, #18212, .T. ) ;
#3683=CARTESIAN_POINT ( 'NONE',  ( -4.773379239211084979, 35.99999999900385461, -19.50000000000000000 ) ) ;
#3689=VERTEX_POINT ( 'NONE', #2428 ) ;
#3692=ORIENTED_EDGE ( 'NONE', *, *, #13223, .F. ) ;
#3694=ORIENTED_EDGE ( 'NONE', *, *, #2933, .T. ) ;
#3702=DIRECTION ( 'NONE',  ( -0.000000000000000000, -1.000000000000000000, -0.000000000000000000 ) ) ;
#3717=VERTEX_POINT ( 'NONE', #2079 ) ;
#3725=CARTESIAN_POINT ( 'NONE',  ( -4.550510256924974684, 36.49999999900384751, -19.00000000000000355 ) ) ;
#3734=EDGE_LOOP ( 'NONE', ( #13710, #6065, #7263, #5551 ) ) ;
#3750=DIRECTION ( 'NONE',  ( 0.000000000000000000, -1.000000000000000000, 0.000000000000000000 ) ) ;
#3769=CARTESIAN_POINT ( 'NONE',  ( -4.990285246489960080, 35.99999999900384751, -25.53533449053936621 ) ) ;
#3770=ADVANCED_FACE ( 'NONE', ( #4182 ), #9611, .F. ) ;
#3776=DIRECTION ( 'NONE',  ( -0.000000000000000000, -0.000000000000000000, 1.000000000000000000 ) ) ;
#3778=DIRECTION ( 'NONE',  ( 1.000000000000000000, 0.000000000000000000, -0.000000000000000000 ) ) ;
#3779=DIRECTION ( 'NONE',  ( 1.000000000000000000, 0.000000000000000000, 0.000000000000000000 ) ) ;
#3789=CARTESIAN_POINT ( 'NONE',  ( 26.45000000029184051, 16.99999999900385461, -26.00000000000000000 ) ) ;
#3793=AXIS2_PLACEMENT_3D ( 'NONE', #22195, #11475, #13490 ) ;
#3815=DIRECTION ( 'NONE',  ( 0.000000000000000000, 0.000000000000000000, 1.000000000000000000 ) ) ;
#3835=PLANE ( 'NONE',  #17895 ) ;
#3852=ORIENTED_EDGE ( 'NONE', *, *, #13872, .T. ) ;
#3863=DIRECTION ( 'NONE',  ( -1.000000000000000000, 0.000000000000000000, 0.000000000000000000 ) ) ;
#3868=CARTESIAN_POINT ( 'NONE',  ( 27.59619407800441948, 27.59619407671642222, -26.50000000000000000 ) ) ;
#3882=ORIENTED_EDGE ( 'NONE', *, *, #22322, .T. ) ;
#3892=CARTESIAN_POINT ( 'NONE',  ( 30.00000000029184832, -0.5000000009961480529, -8.549999999999997158 ) ) ;
#3902=ADVANCED_FACE ( 'NONE', ( #1024, #15701, #20903 ), #6433, .F. ) ;
#3903=LINE ( 'NONE', #7559, #18323 ) ;
#3905=DIRECTION ( 'NONE',  ( 0.000000000000000000, 0.000000000000000000, -1.000000000000000000 ) ) ;
#3910=ORIENTED_EDGE ( 'NONE', *, *, #13856, .F. ) ;
#3917=ORIENTED_EDGE ( 'NONE', *, *, #14247, .F. ) ;
#3931=CARTESIAN_POINT ( 'NONE',  ( 2.918498775983380256E-10, 2.999999999003851503, -19.00000000000000355 ) ) ;
#3945=VECTOR ( 'NONE', #14091, 1000.000000000000000 ) ;
#3947=VECTOR ( 'NONE', #7543, 1000.000000000000000 ) ;
#3970=VERTEX_POINT ( 'NONE', #19477 ) ;
#3971=CARTESIAN_POINT ( 'NONE',  ( -4.239424077913607647, 37.80035007138369707, -28.99269273888553400 ) ) ;
#3973=ORIENTED_EDGE ( 'NONE', *, *, #15996, .F. ) ;
#3981=CYLINDRICAL_SURFACE ( 'NONE', #8672, 0.5000000000000004441 ) ;
#4000=CARTESIAN_POINT ( 'NONE',  ( 36.00000000029184832, 16.99999999900385461, -26.50000000000000000 ) ) ;
#4008=DIRECTION ( 'NONE',  ( 0.000000000000000000, 0.000000000000000000, -1.000000000000000000 ) ) ;
#4043=PLANE ( 'NONE',  #21161 ) ;
#4047=DIRECTION ( 'NONE',  ( 0.000000000000000000, 0.000000000000000000, -1.000000000000000000 ) ) ;
#4064=ORIENTED_EDGE ( 'NONE', *, *, #3386, .T. ) ;
#4066=CARTESIAN_POINT ( 'NONE',  ( 30.00000000029184832, 2.999999999003851503, 0.000000000000000000 ) ) ;
#4070=CARTESIAN_POINT ( 'NONE',  ( 36.00000000029184832, 49.99999999900385461, -28.99999999999999645 ) ) ;
#4073=DIRECTION ( 'NONE',  ( 0.000000000000000000, 0.000000000000000000, -1.000000000000000000 ) ) ;
#4083=CARTESIAN_POINT ( 'NONE',  ( 3.000000000291852764, 42.99999999900385461, -26.00000000000000000 ) ) ;
#4090=VERTEX_POINT ( 'NONE', #2286 ) ;
#4094=DIRECTION ( 'NONE',  ( 1.000000000000000000, 0.000000000000000000, 0.000000000000000000 ) ) ;
#4102=DIRECTION ( 'NONE',  ( 0.000000000000000000, 0.000000000000000000, -1.000000000000000000 ) ) ;
#4111=VERTEX_POINT ( 'NONE', #21947 ) ;
#4114=EDGE_CURVE ( 'NONE', #6361, #19223, #536, .T. ) ;
#4116=CYLINDRICAL_SURFACE ( 'NONE', #9905, 0.5000000000000000000 ) ;
#4130=CARTESIAN_POINT ( 'NONE',  ( -5.623500955413251567, 35.99999999900384751, -19.26867706693546367 ) ) ;
#4142=EDGE_LOOP ( 'NONE', ( #5785, #9358, #4305, #4518 ) ) ;
#4146=( LENGTH_UNIT ( ) NAMED_UNIT ( * ) SI_UNIT ( .MILLI., .METRE. ) );
#4153=DIRECTION ( 'NONE',  ( 0.000000000000000000, 1.000000000000000000, 0.000000000000000000 ) ) ;
#4161=PRODUCT_DEFINITION_CONTEXT ( 'detailed design', #1425, 'design' ) ;
#4168=ORIENTED_EDGE ( 'NONE', *, *, #18622, .T. ) ;
#4177=CARTESIAN_POINT ( 'NONE',  ( -3.999999999708153453, 13.99999999900385106, -22.50000000000000000 ) ) ;
#4180=EDGE_CURVE ( 'NONE', #19813, #3717, #2932, .T. ) ;
#4182=FACE_OUTER_BOUND ( 'NONE', #21170, .T. ) ;
#4191=CARTESIAN_POINT ( 'NONE',  ( -6.056833031243686882, 36.14537244600960264, -28.19628802432849213 ) ) ;
#4209=DIRECTION ( 'NONE',  ( 0.000000000000000000, 0.000000000000000000, -1.000000000000000000 ) ) ;
#4217=AXIS2_PLACEMENT_3D ( 'NONE', #5709, #9805, #13341 ) ;
#4232=VECTOR ( 'NONE', #839, 1000.000000000000114 ) ;
#4233=CARTESIAN_POINT ( 'NONE',  ( -3.499999999708153453, 13.99999999900385106, -19.50000000000000355 ) ) ;
#4249=ORIENTED_EDGE ( 'NONE', *, *, #4767, .F. ) ;
#4252=EDGE_LOOP ( 'NONE', ( #11944, #22444, #10596, #6155, #17967, #15044, #2300 ) ) ;
#4253=AXIS2_PLACEMENT_3D ( 'NONE', #12931, #9289, #12810 ) ;
#4259=AXIS2_PLACEMENT_3D ( 'NONE', #15399, #20841, #832 ) ;
#4260=EDGE_LOOP ( 'NONE', ( #7396, #548, #11338, #11339 ) ) ;
#4264=CARTESIAN_POINT ( 'NONE',  ( 31.55000000029185259, 16.99999999900385461, -29.00000000000000355 ) ) ;
#4265=APPLICATION_CONTEXT ( 'automotive_design' ) ;
#4276=CARTESIAN_POINT ( 'NONE',  ( -5.786576545576798125, 13.89610628501159795, -28.41807078404934117 ) ) ;
#4282=EDGE_LOOP ( 'NONE', ( #11115, #16347, #7593, #7423, #16946, #12824, #19390, #8814, #2392 ) ) ;
#4283=VERTEX_POINT ( 'NONE', #10044 ) ;
#4289=CLOSED_SHELL ( 'NONE', ( #8465, #9973, #6985, #8602, #19738, #3770, #13689, #1432, #21243, #4960, #22507, #1018, #23037, #11307, #2466, #17849, #12289, #11838, #13259, #2732, #22595, #14500, #13541, #13166, #21733, #297, #11117, #12596, #17295, #12566, #20377, #13022, #11507, #7199, #3902, #4908, #1068, #11451, #19510, #7512, #14634, #16823, #15723, #2919, #6579, #9106, #7656, #2691, #12104, #15366, #3636, #21669, #14293, #7936, #14619, #17254, #3094, #19730, #5205, #3003, #15499, #13048, #16557, #12389, #13127, #22608, #11951, #12859, #5337, #10727, #22886, #19996, #12826, #12061, #4769 ) ) ;
#4301=DIRECTION ( 'NONE',  ( 0.000000000000000000, 0.000000000000000000, 1.000000000000000000 ) ) ;
#4305=ORIENTED_EDGE ( 'NONE', *, *, #5455, .F. ) ;
#4314=ORIENTED_EDGE ( 'NONE', *, *, #3651, .T. ) ;
#4336=EDGE_CURVE ( 'NONE', #22242, #283, #17673, .T. ) ;
#4345=EDGE_CURVE ( 'NONE', #18159, #10396, #12611, .T. ) ;
#4347=CARTESIAN_POINT ( 'NONE',  ( -5.784122180648307854, 36.25568647312940840, -16.58536362057690638 ) ) ;
#4358=EDGE_LOOP ( 'NONE', ( #21641, #15913, #7147, #11232 ) ) ;
#4371=LINE ( 'NONE', #10032, #22350 ) ;
#4378=CIRCLE ( 'NONE', #19799, 2.550000000000003819 ) ;
#4379=AXIS2_PLACEMENT_3D ( 'NONE', #9322, #16480, #5806 ) ;
#4393=CIRCLE ( 'NONE', #17545, 0.5000000000000004441 ) ;
#4394=ORIENTED_EDGE ( 'NONE', *, *, #16257, .F. ) ;
#4412=AXIS2_PLACEMENT_3D ( 'NONE', #19853, #10897, #18090 ) ;
#4421=ORIENTED_EDGE ( 'NONE', *, *, #11242, .T. ) ;
#4429=ORIENTED_EDGE ( 'NONE', *, *, #18037, .T. ) ;
#4461=EDGE_CURVE ( 'NONE', #12152, #20279, #1688, .T. ) ;
#4467=FACE_OUTER_BOUND ( 'NONE', #23244, .T. ) ;
#4472=CARTESIAN_POINT ( 'NONE',  ( -3.999999999708153453, 38.99999999900385461, -29.00000000000000355 ) ) ;
#4484=DIRECTION ( 'NONE',  ( -0.7071067811865475727, -0.7071067811865475727, 0.000000000000000000 ) ) ;
#4494=ORIENTED_EDGE ( 'NONE', *, *, #18247, .F. ) ;
#4497=DIRECTION ( 'NONE',  ( 0.000000000000000000, 0.000000000000000000, 1.000000000000000000 ) ) ;
#4518=ORIENTED_EDGE ( 'NONE', *, *, #19272, .F. ) ;
#4539=DIRECTION ( 'NONE',  ( -1.000000000000000000, 0.000000000000000000, -1.613696256722611405E-16 ) ) ;
#4543=VERTEX_POINT ( 'NONE', #11196 ) ;
#4544=CARTESIAN_POINT ( 'NONE',  ( 36.00000000029184832, 2.999999999003851503, 0.000000000000000000 ) ) ;
#4548=EDGE_LOOP ( 'NONE', ( #22260, #9674, #11119, #9817 ) ) ;
#4557=CARTESIAN_POINT ( 'NONE',  ( -6.977878452303022172, 35.99999999900387593, -18.50953884562097684 ) ) ;
#4561=LINE ( 'NONE', #20933, #13811 ) ;
#4567=VERTEX_POINT ( 'NONE', #9438 ) ;
#4578=LINE ( 'NONE', #7659, #22137 ) ;
#4584=DIRECTION ( 'NONE',  ( -0.000000000000000000, 1.000000000000000000, -0.000000000000000000 ) ) ;
#4590=DIRECTION ( 'NONE',  ( -0.000000000000000000, -1.000000000000000000, -0.000000000000000000 ) ) ;
#4607=ORIENTED_EDGE ( 'NONE', *, *, #13156, .T. ) ;
#4615=AXIS2_PLACEMENT_3D ( 'NONE', #993, #762, #6050 ) ;
#4639=ORIENTED_EDGE ( 'NONE', *, *, #4114, .T. ) ;
#4642=EDGE_CURVE ( 'NONE', #22761, #4543, #9287, .T. ) ;
#4648=EDGE_CURVE ( 'NONE', #20913, #283, #1027, .T. ) ;
#4667=LINE ( 'NONE', #6208, #327 ) ;
#4682=EDGE_CURVE ( 'NONE', #20043, #17223, #22435, .T. ) ;
#4685=CARTESIAN_POINT ( 'NONE',  ( -4.711587335155682510, 35.99999999900384751, -19.05331844708923938 ) ) ;
#4697=DIRECTION ( 'NONE',  ( 0.000000000000000000, 0.000000000000000000, -1.000000000000000000 ) ) ;
#4703=ORIENTED_EDGE ( 'NONE', *, *, #4336, .F. ) ;
#4706=CARTESIAN_POINT ( 'NONE',  ( 31.55000000029185259, 16.99999999900385461, -19.00000000000000355 ) ) ;
#4707=EDGE_CURVE ( 'NONE', #688, #690, #15838, .T. ) ;
#4714=CARTESIAN_POINT ( 'NONE',  ( 29.00000000029184832, 16.99999999900385461, -26.50000000000000000 ) ) ;
#4721=ORIENTED_EDGE ( 'NONE', *, *, #15102, .T. ) ;
#4751=ORIENTED_EDGE ( 'NONE', *, *, #4707, .F. ) ;
#4760=LINE ( 'NONE', #6071, #20798 ) ;
#4761=VERTEX_POINT ( 'NONE', #4472 ) ;
#4767=EDGE_CURVE ( 'NONE', #16772, #2264, #2461, .T. ) ;
#4769=ADVANCED_FACE ( 'NONE', ( #21277 ), #9775, .F. ) ;
#4779=ORIENTED_EDGE ( 'NONE', *, *, #1648, .T. ) ;
#4798=EDGE_CURVE ( 'NONE', #1665, #14963, #13002, .T. ) ;
#4803=DIRECTION ( 'NONE',  ( 0.000000000000000000, 0.000000000000000000, -1.000000000000000000 ) ) ;
#4811=ORIENTED_EDGE ( 'NONE', *, *, #2623, .T. ) ;
#4813=VECTOR ( 'NONE', #17382, 1000.000000000000000 ) ;
#4833=AXIS2_PLACEMENT_3D ( 'NONE', #14063, #21484, #16044 ) ;
#4837=ORIENTED_EDGE ( 'NONE', *, *, #204, .F. ) ;
#4841=ORIENTED_EDGE ( 'NONE', *, *, #21449, .T. ) ;
#4846=LINE ( 'NONE', #15658, #8722 ) ;
#4871=VERTEX_POINT ( 'NONE', #3725 ) ;
#4875=LINE ( 'NONE', #8647, #14380 ) ;
#4879=PLANE ( 'NONE',  #9626 ) ;
#4895=CARTESIAN_POINT ( 'NONE',  ( 2.918498775983380256E-10, 2.999999999003851503, -32.00000000000000000 ) ) ;
#4896=ORIENTED_EDGE ( 'NONE', *, *, #16010, .T. ) ;
#4902=CARTESIAN_POINT ( 'NONE',  ( -6.566827241915921043, 35.99999999896398606, -18.68676989095779462 ) ) ;
#4908=ADVANCED_FACE ( 'NONE', ( #14784, #1952, #3620 ), #3835, .F. ) ;
#4911=DIRECTION ( 'NONE',  ( -1.000000000000000000, -0.000000000000000000, 0.000000000000000000 ) ) ;
#4917=ORIENTED_EDGE ( 'NONE', *, *, #13149, .T. ) ;
#4919=CARTESIAN_POINT ( 'NONE',  ( -4.550510256924973795, 35.99999999900384751, -25.99999999999999645 ) ) ;
#4926=VERTEX_POINT ( 'NONE', #18656 ) ;
#4928=CARTESIAN_POINT ( 'NONE',  ( -5.549486778973212076, 36.19267127072036772, -26.13446119014969327 ) ) ;
#4931=CIRCLE ( 'NONE', #21086, 5.999999999999998224 ) ;
#4935=PLANE ( 'NONE',  #1276 ) ;
#4943=CARTESIAN_POINT ( 'NONE',  ( 0.000000000000000000, 0.000000000000000000, 0.000000000000000000 ) ) ;
#4946=VECTOR ( 'NONE', #11352, 1000.000000000000000 ) ;
#4948=ORIENTED_EDGE ( 'NONE', *, *, #17273, .T. ) ;
#4949=ORIENTED_EDGE ( 'NONE', *, *, #6064, .T. ) ;
#4952=ORIENTED_EDGE ( 'NONE', *, *, #6231, .F. ) ;
#4959=DIRECTION ( 'NONE',  ( -0.000000000000000000, -0.000000000000000000, 1.000000000000000000 ) ) ;
#4960=ADVANCED_FACE ( 'NONE', ( #19016, #22778, #8651 ), #4879, .F. ) ;
#4965=AXIS2_PLACEMENT_3D ( 'NONE', #3470, #10980, #5475 ) ;
#4973=DIRECTION ( 'NONE',  ( 0.000000000000000000, 0.000000000000000000, -1.000000000000000000 ) ) ;
#4981=EDGE_CURVE ( 'NONE', #22384, #11457, #12507, .T. ) ;
#4982=ORIENTED_EDGE ( 'NONE', *, *, #21771, .F. ) ;
#4984=CIRCLE ( 'NONE', #4217, 2.549999999999998934 ) ;
#4988=VECTOR ( 'NONE', #19084, 1000.000000000000000 ) ;
#4989=ORIENTED_EDGE ( 'NONE', *, *, #1153, .F. ) ;
#4998=DIRECTION ( 'NONE',  ( 1.000000000000000000, 0.000000000000000000, 0.000000000000000000 ) ) ;
#5002=CARTESIAN_POINT ( 'NONE',  ( -6.999999999708143683, 13.99999999900385106, -18.79789498886801624 ) ) ;
#5009=DIRECTION ( 'NONE',  ( -0.7071067811865474617, 0.7071067811865474617, -0.000000000000000000 ) ) ;
#5021=CIRCLE ( 'NONE', #15163, 7.000000000000000000 ) ;
#5033=CARTESIAN_POINT ( 'NONE',  ( 30.00000000029184832, -0.5000000009961480529, -5.999999999999998224 ) ) ;
#5047=CARTESIAN_POINT ( 'NONE',  ( -5.273209981518101053, 36.26961333663654585, -26.07660499612833149 ) ) ;
#5091=CARTESIAN_POINT ( 'NONE',  ( 35.50000000029184832, -9.961476088449217059E-10, -18.50000000000000355 ) ) ;
#5093=CARTESIAN_POINT ( 'NONE',  ( -3.999999999708153453, 35.99999999900384751, -19.50000000000000355 ) ) ;
#5101=DIRECTION ( 'NONE',  ( -1.000000000000000000, 0.000000000000000000, 0.000000000000000000 ) ) ;
#5112=AXIS2_PLACEMENT_3D ( 'NONE', #16355, #256, #8854 ) ;
#5150=DIRECTION ( 'NONE',  ( 0.000000000000000000, 1.000000000000000000, -0.000000000000000000 ) ) ;
#5152=CARTESIAN_POINT ( 'NONE',  ( -6.999999999708142795, 49.99999999900385461, -18.99999999999998934 ) ) ;
#5159=AXIS2_PLACEMENT_3D ( 'NONE', #10452, #23168, #9036 ) ;
#5166=CARTESIAN_POINT ( 'NONE',  ( -6.605954977387137994, 35.99999999900384751, -26.25080446718044414 ) ) ;
#5205=ADVANCED_FACE ( 'NONE', ( #5839 ), #18517, .T. ) ;
#5208=ORIENTED_EDGE ( 'NONE', *, *, #13317, .F. ) ;
#5220=CARTESIAN_POINT ( 'NONE',  ( 36.00000000029184832, -9.961476088449217059E-10, -45.00000000000000000 ) ) ;
#5222=CARTESIAN_POINT ( 'NONE',  ( -3.999999999708139686, 49.99999999900386172, -15.99999999999999289 ) ) ;
#5233=AXIS2_PLACEMENT_3D ( 'NONE', #21953, #5845, #9127 ) ;
#5235=VERTEX_POINT ( 'NONE', #12998 ) ;
#5255=CARTESIAN_POINT ( 'NONE',  ( -5.454524251050746564, 13.82936183575430356, -16.36878710987171459 ) ) ;
#5261=EDGE_LOOP ( 'NONE', ( #6533, #2353, #5464, #4064 ) ) ;
#5272=AXIS2_PLACEMENT_3D ( 'NONE', #6425, #1016, #14916 ) ;
#5286=CARTESIAN_POINT ( 'NONE',  ( -6.231825765894918767, 35.99999999900384751, -26.01458861726397487 ) ) ;
#5293=ORIENTED_EDGE ( 'NONE', *, *, #6066, .F. ) ;
#5306=DIRECTION ( 'NONE',  ( 1.000000000000000000, 0.000000000000000000, 0.000000000000000000 ) ) ;
#5317=CARTESIAN_POINT ( 'NONE',  ( -4.550510256924974684, 35.99999999900384751, -25.50000000000000000 ) ) ;
#5319=FACE_OUTER_BOUND ( 'NONE', #12052, .T. ) ;
#5328=EDGE_CURVE ( 'NONE', #3083, #8469, #12479, .T. ) ;
#5330=CARTESIAN_POINT ( 'NONE',  ( 35.50000000029184832, 2.999999999003851503, -26.00000000000000000 ) ) ;
#5334=DIRECTION ( 'NONE',  ( 0.000000000000000000, -1.000000000000000000, 0.000000000000000000 ) ) ;
#5336=ORIENTED_EDGE ( 'NONE', *, *, #21222, .F. ) ;
#5337=ADVANCED_FACE ( 'NONE', ( #996 ), #20760, .F. ) ;
#5356=CYLINDRICAL_SURFACE ( 'NONE', #15392, 2.550000000000002043 ) ;
#5359=FACE_OUTER_BOUND ( 'NONE', #22387, .T. ) ;
#5366=CARTESIAN_POINT ( 'NONE',  ( -5.281014309470091206, 13.78823385074812613, -16.28034847426729925 ) ) ;
#5372=CARTESIAN_POINT ( 'NONE',  ( 2.918498775983380256E-10, 2.999999999003851503, -32.00000000000000000 ) ) ;
#5439=AXIS2_PLACEMENT_3D ( 'NONE', #260, #13192, #7774 ) ;
#5444=AXIS2_PLACEMENT_3D ( 'NONE', #22157, #754, #7806 ) ;
#5448=CARTESIAN_POINT ( 'NONE',  ( 6.000000000291855429, -9.961476088449217059E-10, -36.44999999999999574 ) ) ;
#5455=EDGE_CURVE ( 'NONE', #10365, #16744, #21511, .T. ) ;
#5457=AXIS2_PLACEMENT_3D ( 'NONE', #21658, #19531, #3310 ) ;
#5464=ORIENTED_EDGE ( 'NONE', *, *, #2608, .F. ) ;
#5471=AXIS2_PLACEMENT_3D ( 'NONE', #5033, #10559, #12315 ) ;
#5475=DIRECTION ( 'NONE',  ( 0.7071067811865475727, 0.7071067811865475727, 0.000000000000000000 ) ) ;
#5486=EDGE_CURVE ( 'NONE', #14699, #1834, #21801, .T. ) ;
#5489=ORIENTED_EDGE ( 'NONE', *, *, #10925, .T. ) ;
#5490=ORIENTED_EDGE ( 'NONE', *, *, #15626, .F. ) ;
#5507=DIRECTION ( 'NONE',  ( 0.7071067811865474617, -0.7071067811865474617, 0.000000000000000000 ) ) ;
#5541=DIRECTION ( 'NONE',  ( 0.000000000000000000, 0.000000000000000000, -1.000000000000000000 ) ) ;
#5551=ORIENTED_EDGE ( 'NONE', *, *, #22752, .F. ) ;
#5554=LINE ( 'NONE', #376, #1325 ) ;
#5560=AXIS2_PLACEMENT_3D ( 'NONE', #12146, #5334, #19336 ) ;
#5563=CARTESIAN_POINT ( 'NONE',  ( -6.999999999708142795, 49.99999999900385461, -18.99999999999998934 ) ) ;
#5570=CIRCLE ( 'NONE', #14579, 6.500000000000000888 ) ;
#5571=CARTESIAN_POINT ( 'NONE',  ( 33.59619407800440882, 21.59619407671641866, -26.50000000000000000 ) ) ;
#5574=EDGE_CURVE ( 'NONE', #19243, #12740, #7898, .T. ) ;
#5576=B_SPLINE_CURVE_WITH_KNOTS ( 'NONE', 3,
 ( #7221, #12735, #10956, #4130, #2025, #9211, #3683, #14385 ),
 .UNSPECIFIED., .F., .F.,
 ( 4, 2, 2, 4 ),
 ( 2.405267759940038380E-17, 0.001312337235399278637, 0.001968505853098905922, 0.002624674470798532989 ),
 .UNSPECIFIED. ) ;
#5582=ORIENTED_EDGE ( 'NONE', *, *, #17415, .F. ) ;
#5592=VECTOR ( 'NONE', #18237, 1000.000000000000000 ) ;
#5599=CARTESIAN_POINT ( 'NONE',  ( -6.999999999708142795, 38.99999999900385461, -26.50000000000000000 ) ) ;
#5616=EDGE_CURVE ( 'NONE', #10396, #14621, #14003, .T. ) ;
#5617=DIRECTION ( 'NONE',  ( 0.000000000000000000, -1.000000000000000000, 0.000000000000000000 ) ) ;
#5622=CIRCLE ( 'NONE', #12745, 0.5000000000000004441 ) ;
#5641=CARTESIAN_POINT ( 'NONE',  ( -6.147973203409447862, 36.05667699661075432, -18.72569195403428566 ) ) ;
#5650=B_SPLINE_CURVE_WITH_KNOTS ( 'NONE', 3,
 ( #20340, #16337, #21656, #21768 ),
 .UNSPECIFIED., .F., .F.,
 ( 4, 4 ),
 ( 0.000000000000000000, 1.361771040838494909E-05 ),
 .UNSPECIFIED. ) ;
#5675=AXIS2_PLACEMENT_3D ( 'NONE', #3068, #13772, #1534 ) ;
#5679=CARTESIAN_POINT ( 'NONE',  ( -6.917363703046245149, 36.00086243655339757, -18.25935642526717828 ) ) ;
#5700=EDGE_LOOP ( 'NONE', ( #17127, #2973, #23154, #14138, #12358, #8466, #22562, #15427, #1103 ) ) ;
#5703=VERTEX_POINT ( 'NONE', #17173 ) ;
#5709=CARTESIAN_POINT ( 'NONE',  ( 30.00000000029184832, 2.999999999003851503, -5.999999999999998224 ) ) ;
#5719=ORIENTED_EDGE ( 'NONE', *, *, #1628, .F. ) ;
#5722=VERTEX_POINT ( 'NONE', #13777 ) ;
#5729=ORIENTED_EDGE ( 'NONE', *, *, #4767, .T. ) ;
#5744=CARTESIAN_POINT ( 'NONE',  ( 2.918498775983380256E-10, -9.961476088449217059E-10, -45.00000000000000000 ) ) ;
#5754=VECTOR ( 'NONE', #3776, 1000.000000000000000 ) ;
#5765=FACE_OUTER_BOUND ( 'NONE', #4548, .T. ) ;
#5771=CARTESIAN_POINT ( 'NONE',  ( -3.999999999708153453, 35.99999999900384751, -26.50000000000000000 ) ) ;
#5777=AXIS2_PLACEMENT_3D ( 'NONE', #5563, #3779, #261 ) ;
#5783=ORIENTED_EDGE ( 'NONE', *, *, #13872, .F. ) ;
#5785=ORIENTED_EDGE ( 'NONE', *, *, #22142, .F. ) ;
#5795=AXIS2_PLACEMENT_3D ( 'NONE', #11725, #9856, #9747 ) ;
#5806=DIRECTION ( 'NONE',  ( 0.000000000000000000, 0.000000000000000000, -1.000000000000000000 ) ) ;
#5818=UNCERTAINTY_MEASURE_WITH_UNIT (LENGTH_MEASURE( 1.000000000000000082E-05 ), #4146, 'distance_accuracy_value', 'NONE');
#5825=VERTEX_POINT ( 'NONE', #14244 ) ;
#5831=EDGE_CURVE ( 'NONE', #3520, #14012, #19887, .T. ) ;
#5836=AXIS2_PLACEMENT_3D ( 'NONE', #12476, #19669, #21674 ) ;
#5839=FACE_OUTER_BOUND ( 'NONE', #13270, .T. ) ;
#5843=ORIENTED_EDGE ( 'NONE', *, *, #17863, .F. ) ;
#5845=DIRECTION ( 'NONE',  ( -1.000000000000000000, 0.000000000000000000, -1.613696256722611405E-16 ) ) ;
#5863=DIRECTION ( 'NONE',  ( 1.000000000000000000, 0.000000000000000000, 0.000000000000000000 ) ) ;
#5877=CARTESIAN_POINT ( 'NONE',  ( -4.499999999708154341, 35.49999999900384751, -26.00000000000000000 ) ) ;
#5879=DIRECTION ( 'NONE',  ( 1.000000000000000000, 0.000000000000000000, 0.000000000000000000 ) ) ;
#5880=CIRCLE ( 'NONE', #603, 2.550000000000003819 ) ;
#5887=PLANE ( 'NONE',  #8957 ) ;
#5895=CARTESIAN_POINT ( 'NONE',  ( 36.00000000029184832, 2.999999999003851503, -26.50000000000000000 ) ) ;
#5922=AXIS2_PLACEMENT_3D ( 'NONE', #3868, #21659, #7413 ) ;
#5928=ORIENTED_EDGE ( 'NONE', *, *, #17152, .F. ) ;
#5946=DIRECTION ( 'NONE',  ( 0.000000000000000000, 0.000000000000000000, -1.000000000000000000 ) ) ;
#5952=AXIS2_PLACEMENT_3D ( 'NONE', #20695, #2810, #9987 ) ;
#5967=EDGE_CURVE ( 'NONE', #5722, #16629, #11051, .T. ) ;
#5972=( BOUNDED_SURFACE ( )  B_SPLINE_SURFACE ( 3, 2, ( 
 ( #21058, #4919, #12327 ),
 ( #12085, #5, #12571 ),
 ( #21417, #21178, #10460 ),
 ( #15850, #19278, #5047 ),
 ( #12206, #3525, #23061 ),
 ( #5286, #10689, #14104 ),
 ( #5166, #19517, #12446 ),
 ( #10570, #17873, #8932 ) ),
 .UNSPECIFIED., .F., .F., .F. ) 
 B_SPLINE_SURFACE_WITH_KNOTS ( ( 4, 2, 2, 4 ),
 ( 3, 3 ),
 ( 0.000000000000000000, 0.0006647103312144571167, 0.001329420662428914233, 0.002658841324857828467 ),
 ( 0.000000000000000000, 1.000000000000000000 ),
 .UNSPECIFIED. ) 
 GEOMETRIC_REPRESENTATION_ITEM ( )  RATIONAL_B_SPLINE_SURFACE ( (
 ( 1.000000000000000000, 0.7071067811865475727, 1.000000000000000000),
 ( 1.000000000000000000, 0.7467694970713046887, 1.000000000000000000),
 ( 1.000000000000000000, 0.7847899295822856613, 1.000000000000000000),
 ( 1.000000000000000000, 0.8553546080387325334, 1.000000000000000000),
 ( 1.000000000000000000, 0.8874277420052644194, 1.000000000000000000),
 ( 1.000000000000000000, 0.9672515829027974466, 1.000000000000000000),
 ( 1.000000000000000000, 0.9993132011596692621, 1.000000000000000000),
 ( 1.000000000000000000, 0.9999716904335731460, 1.000000000000000000) ) ) 
 REPRESENTATION_ITEM ( '' )  SURFACE ( )  );
#5982=EDGE_LOOP ( 'NONE', ( #8056, #23209, #20708, #18839, #3694, #10773, #7937 ) ) ;
#5983=VERTEX_POINT ( 'NONE', #11506 ) ;
#6022=CYLINDRICAL_SURFACE ( 'NONE', #10592, 0.5000000000000004441 ) ;
#6043=ORIENTED_EDGE ( 'NONE', *, *, #10672, .F. ) ;
#6050=DIRECTION ( 'NONE',  ( 0.000000000000000000, 0.000000000000000000, 1.000000000000000000 ) ) ;
#6056=AXIS2_PLACEMENT_3D ( 'NONE', #6476, #11525, #15405 ) ;
#6064=EDGE_CURVE ( 'NONE', #8658, #5235, #3340, .T. ) ;
#6065=ORIENTED_EDGE ( 'NONE', *, *, #3421, .T. ) ;
#6066=EDGE_CURVE ( 'NONE', #4871, #14655, #14218, .T. ) ;
#6071=CARTESIAN_POINT ( 'NONE',  ( 5.550000000291854363, 42.99999999900385461, -19.49999999999998934 ) ) ;
#6085=FACE_BOUND ( 'NONE', #14559, .T. ) ;
#6106=CIRCLE ( 'NONE', #18860, 2.550000000000003819 ) ;
#6134=CARTESIAN_POINT ( 'NONE',  ( -5.688936712956111919, 36.29949271875472050, -16.51803887880629418 ) ) ;
#6153=EDGE_CURVE ( 'NONE', #5825, #12740, #23208, .T. ) ;
#6155=ORIENTED_EDGE ( 'NONE', *, *, #19160, .T. ) ;
#6157=EDGE_LOOP ( 'NONE', ( #8519, #15394, #9567, #19174 ) ) ;
#6170=CARTESIAN_POINT ( 'NONE',  ( 2.918498775983380256E-10, 2.999999999003851503, -45.00000000000000000 ) ) ;
#6175=FACE_OUTER_BOUND ( 'NONE', #22386, .T. ) ;
#6177=VECTOR ( 'NONE', #3778, 1000.000000000000000 ) ;
#6189=ORIENTED_EDGE ( 'NONE', *, *, #16707, .T. ) ;
#6190=DIRECTION ( 'NONE',  ( 1.000000000000000000, 0.000000000000000000, 0.000000000000000000 ) ) ;
#6194=ORIENTED_EDGE ( 'NONE', *, *, #6670, .T. ) ;
#6199=CARTESIAN_POINT ( 'NONE',  ( 36.00000000029184832, 49.99999999900385461, -16.00000000000000000 ) ) ;
#6208=CARTESIAN_POINT ( 'NONE',  ( 6.000000000291855429, -0.5000000009961480529, -3.449999999999997957 ) ) ;
#6213=EDGE_LOOP ( 'NONE', ( #22947, #10578, #15601 ) ) ;
#6225=CARTESIAN_POINT ( 'NONE',  ( -6.083292711304078892, 36.06725630338318211, -18.74270568520632807 ) ) ;
#6231=EDGE_CURVE ( 'NONE', #8964, #19696, #17984, .T. ) ;
#6233=DIRECTION ( 'NONE',  ( 0.000000000000000000, -1.000000000000000000, 0.000000000000000000 ) ) ;
#6237=ORIENTED_EDGE ( 'NONE', *, *, #5328, .T. ) ;
#6241=EDGE_CURVE ( 'NONE', #8991, #8964, #15343, .T. ) ;
#6273=LINE ( 'NONE', #984, #4988 ) ;
#6282=PLANE ( 'NONE',  #20844 ) ;
#6293=CARTESIAN_POINT ( 'NONE',  ( -6.587771436282945814, 13.98878796535109359, -27.53104552455945608 ) ) ;
#6310=VECTOR ( 'NONE', #12493, 1000.000000000000000 ) ;
#6322=ORIENTED_EDGE ( 'NONE', *, *, #19, .F. ) ;
#6352=CIRCLE ( 'NONE', #9356, 6.500000000000005329 ) ;
#6361=VERTEX_POINT ( 'NONE', #22402 ) ;
#6394=DIRECTION ( 'NONE',  ( 0.000000000000000000, 0.000000000000000000, -1.000000000000000000 ) ) ;
#6397=PRESENTATION_STYLE_ASSIGNMENT (( #2624 ) ) ;
#6409=CARTESIAN_POINT ( 'NONE',  ( -6.999999999708145459, 13.99999999900385106, -26.20210501113198376 ) ) ;
#6419=ORIENTED_EDGE ( 'NONE', *, *, #18305, .F. ) ;
#6424=ORIENTED_EDGE ( 'NONE', *, *, #2608, .T. ) ;
#6425=CARTESIAN_POINT ( 'NONE',  ( -3.999999999708153453, 35.99999999900384751, -15.50000000000000000 ) ) ;
#6427=DIRECTION ( 'NONE',  ( -1.000000000000000000, 0.000000000000000000, 0.000000000000000000 ) ) ;
#6433=PLANE ( 'NONE',  #2216 ) ;
#6464=CARTESIAN_POINT ( 'NONE',  ( 33.94974746859769255, 21.94974746730969528, -15.99999999999999289 ) ) ;
#6468=CIRCLE ( 'NONE', #18488, 2.999999999999999112 ) ;
#6476=CARTESIAN_POINT ( 'NONE',  ( 30.00000000029184832, -9.961476088449217059E-10, -39.00000000000000000 ) ) ;
#6485=EDGE_CURVE ( 'NONE', #8753, #4567, #2161, .T. ) ;
#6502=CARTESIAN_POINT ( 'NONE',  ( -4.550510256924974684, 36.49999999900384751, -19.50000000000000355 ) ) ;
#6505=EDGE_CURVE ( 'NONE', #20279, #22431, #23229, .T. ) ;
#6527=VECTOR ( 'NONE', #17522, 1000.000000000000000 ) ;
#6533=ORIENTED_EDGE ( 'NONE', *, *, #17152, .T. ) ;
#6538=EDGE_CURVE ( 'NONE', #2294, #13206, #17319, .T. ) ;
#6547=FACE_OUTER_BOUND ( 'NONE', #12234, .T. ) ;
#6555=CARTESIAN_POINT ( 'NONE',  ( 2.918498775983380256E-10, 5.999999999003851059, -15.99999999999999289 ) ) ;
#6564=EDGE_LOOP ( 'NONE', ( #20540, #1234, #5843, #20194, #6424, #9621 ) ) ;
#6569=ORIENTED_EDGE ( 'NONE', *, *, #5328, .F. ) ;
#6574=CARTESIAN_POINT ( 'NONE',  ( 3.000000000291852764, 42.99999999900385461, -19.00000000000000355 ) ) ;
#6577=CARTESIAN_POINT ( 'NONE',  ( 36.00000000029184832, 2.999999999003851503, -32.00000000000000000 ) ) ;
#6579=ADVANCED_FACE ( 'NONE', ( #15565 ), #8287, .T. ) ;
#6606=ORIENTED_EDGE ( 'NONE', *, *, #17536, .T. ) ;
#6617=DIRECTION ( 'NONE',  ( -1.000000000000000000, -0.000000000000000000, -0.000000000000000000 ) ) ;
#6639=B_SPLINE_CURVE_WITH_KNOTS ( 'NONE', 3,
 ( #5317, #16006, #3769, #3326, #21328, #15884, #3437, #1780 ),
 .UNSPECIFIED., .F., .F.,
 ( 4, 2, 2, 4 ),
 ( 0.000000000000000000, 0.0006592848877641304360, 0.001318569775528260872, 0.002637139551056521744 ),
 .UNSPECIFIED. ) ;
#6643=FACE_OUTER_BOUND ( 'NONE', #866, .T. ) ;
#6648=CARTESIAN_POINT ( 'NONE',  ( 6.000000000291855429, 2.999999999003851503, -3.449999999999997957 ) ) ;
#6670=EDGE_CURVE ( 'NONE', #22761, #178, #3903, .T. ) ;
#6676=( BOUNDED_SURFACE ( )  B_SPLINE_SURFACE ( 3, 2, ( 
 ( #11616, #8100, #15612 ),
 ( #7980, #4685, #19147 ),
 ( #22567, #15151, #18806 ),
 ( #6684, #10099, #13628 ),
 ( #9863, #19257, #22343 ),
 ( #6225, #11858, #18926 ),
 ( #21041, #4902, #9753 ),
 ( #2679, #4557, #16904 ) ),
 .UNSPECIFIED., .F., .F., .T. ) 
 B_SPLINE_SURFACE_WITH_KNOTS ( ( 4, 2, 2, 4 ),
 ( 3, 3 ),
 ( 1.409462824231155764E-18, 0.0006647103312235273353, 0.001329420662447053370, 0.002658841324894105438 ),
 ( 0.000000000000000000, 1.000000000000000000 ),
 .UNSPECIFIED. ) 
 GEOMETRIC_REPRESENTATION_ITEM ( )  RATIONAL_B_SPLINE_SURFACE ( (
 ( 1.000000000000000000, 0.7071067811865475727, 1.000000000000000000),
 ( 1.000000000000000000, 0.7467694970717694281, 1.000000000000000000),
 ( 1.000000000000000000, 0.7847899295834248612, 1.000000000000000000),
 ( 1.000000000000000000, 0.8553546080404790253, 1.000000000000000000),
 ( 1.000000000000000000, 0.8874277420076976952, 1.000000000000000000),
 ( 1.000000000000000000, 0.9672515829044651126, 1.000000000000000000),
 ( 1.000000000000000000, 0.9993132011618868216, 1.000000000000000000),
 ( 1.000000000000000000, 0.9999716904336592993, 1.000000000000000000) ) ) 
 REPRESENTATION_ITEM ( '' )  SURFACE ( )  );
#6682=AXIS2_PLACEMENT_3D ( 'NONE', #5571, #20146, #166 ) ;
#6684=CARTESIAN_POINT ( 'NONE',  ( -5.273209981528717449, 36.26961333663339815, -18.92339500386973938 ) ) ;
#6694=FACE_OUTER_BOUND ( 'NONE', #17932, .T. ) ;
#6695=DIRECTION ( 'NONE',  ( 1.000000000000000000, 0.000000000000000000, 0.000000000000000000 ) ) ;
#6704=VECTOR ( 'NONE', #3702, 1000.000000000000000 ) ;
#6710=CARTESIAN_POINT ( 'NONE',  ( -6.959810536856680940, 36.00015702695179698, -26.48940942388196618 ) ) ;
#6731=ORIENTED_EDGE ( 'NONE', *, *, #1058, .T. ) ;
#6734=CYLINDRICAL_SURFACE ( 'NONE', #9532, 2.550000000000000711 ) ;
#6741=CIRCLE ( 'NONE', #17257, 5.999999999999998224 ) ;
#6743=CARTESIAN_POINT ( 'NONE',  ( -3.499999999708153453, 2.999999999003851503, -25.50000000000000000 ) ) ;
#6752=VERTEX_POINT ( 'NONE', #16586 ) ;
#6774=CARTESIAN_POINT ( 'NONE',  ( -6.979783269036462734, 14.00008466144083030, -18.59869175759557791 ) ) ;
#6776=DIRECTION ( 'NONE',  ( 1.858632295689435609E-16, 1.000000000000000000, -0.000000000000000000 ) ) ;
#6779=EDGE_CURVE ( 'NONE', #1430, #14170, #2258, .T. ) ;
#6806=LINE ( 'NONE', #13974, #13013 ) ;
#6823=CARTESIAN_POINT ( 'NONE',  ( -3.499999999708153453, 35.49999999900384751, -19.00000000000000355 ) ) ;
#6826=CARTESIAN_POINT ( 'NONE',  ( 2.918498775983380256E-10, 6.999999999003851947, -19.00000000000000355 ) ) ;
#6831=FACE_OUTER_BOUND ( 'NONE', #3114, .T. ) ;
#6863=AXIS2_PLACEMENT_3D ( 'NONE', #17343, #16878, #3010 ) ;
#6896=CIRCLE ( 'NONE', #14022, 2.549999999999998490 ) ;
#6898=CARTESIAN_POINT ( 'NONE',  ( 6.000000000291855429, -0.5000000009961480529, -41.55000000000000426 ) ) ;
#6915=FACE_OUTER_BOUND ( 'NONE', #15602, .T. ) ;
#6921=CARTESIAN_POINT ( 'NONE',  ( 36.00000000029184832, 5.999999999003851059, -16.00000000000000000 ) ) ;
#6949=CARTESIAN_POINT ( 'NONE',  ( -4.550510256924974684, 36.49999999900384751, -26.00000000000000000 ) ) ;
#6959=EDGE_CURVE ( 'NONE', #22269, #1665, #13082, .T. ) ;
#6984=FACE_OUTER_BOUND ( 'NONE', #3734, .T. ) ;
#6985=ADVANCED_FACE ( 'NONE', ( #12466 ), #7313, .F. ) ;
#6996=FACE_OUTER_BOUND ( 'NONE', #18198, .T. ) ;
#7000=AXIS2_PLACEMENT_3D ( 'NONE', #13965, #1510, #14090 ) ;
#7034=ORIENTED_EDGE ( 'NONE', *, *, #16111, .F. ) ;
#7041=CARTESIAN_POINT ( 'NONE',  ( 30.00000000029184832, 2.999999999003851503, -5.999999999999998224 ) ) ;
#7046=FACE_OUTER_BOUND ( 'NONE', #22941, .T. ) ;
#7077=FACE_OUTER_BOUND ( 'NONE', #2675, .T. ) ;
#7099=MECHANICAL_DESIGN_GEOMETRIC_PRESENTATION_REPRESENTATION('',(#2189),#20993);
#7100=FACE_OUTER_BOUND ( 'NONE', #12473, .T. ) ;
#7101=DIRECTION ( 'NONE',  ( 0.000000000000000000, 0.000000000000000000, 1.000000000000000000 ) ) ;
#7128=ORIENTED_EDGE ( 'NONE', *, *, #4345, .F. ) ;
#7147=ORIENTED_EDGE ( 'NONE', *, *, #11533, .T. ) ;
#7172=ORIENTED_EDGE ( 'NONE', *, *, #12685, .T. ) ;
#7182=ORIENTED_EDGE ( 'NONE', *, *, #16611, .F. ) ;
#7188=FACE_OUTER_BOUND ( 'NONE', #2756, .T. ) ;
#7199=ADVANCED_FACE ( 'NONE', ( #7645, #14819, #22000 ), #5887, .F. ) ;
#7204=CARTESIAN_POINT ( 'NONE',  ( -3.499999999708153453, 38.99999999900385461, -26.00000000000000000 ) ) ;
#7207=DIRECTION ( 'NONE',  ( 1.000000000000000000, 0.000000000000000000, 0.000000000000000000 ) ) ;
#7210=CARTESIAN_POINT ( 'NONE',  ( 31.55000000029185259, 16.99999999900385461, -19.49999999999998934 ) ) ;
#7211=CARTESIAN_POINT ( 'NONE',  ( 36.00000000029184832, 16.99999999900385461, -29.00000000000000355 ) ) ;
#7217=DIRECTION ( 'NONE',  ( -0.000000000000000000, 1.000000000000000000, -0.000000000000000000 ) ) ;
#7220=AXIS2_PLACEMENT_3D ( 'NONE', #22975, #14143, #11158 ) ;
#7221=CARTESIAN_POINT ( 'NONE',  ( -6.962001439796694058, 35.99999999900384751, -18.52402997057235723 ) ) ;
#7223=VERTEX_POINT ( 'NONE', #6464 ) ;
#7240=AXIS2_PLACEMENT_3D ( 'NONE', #7041, #12191, #3276 ) ;
#7246=EDGE_CURVE ( 'NONE', #15368, #12647, #17034, .T. ) ;
#7250=CARTESIAN_POINT ( 'NONE',  ( 26.45000000029184051, 16.99999999900385461, -25.50000000000000355 ) ) ;
#7263=ORIENTED_EDGE ( 'NONE', *, *, #17401, .T. ) ;
#7313=CYLINDRICAL_SURFACE ( 'NONE', #9713, 2.550000000000002043 ) ;
#7330=FACE_OUTER_BOUND ( 'NONE', #16832, .T. ) ;
#7331=DIRECTION ( 'NONE',  ( 0.000000000000000000, 0.000000000000000000, 1.000000000000000000 ) ) ;
#7367=CARTESIAN_POINT ( 'NONE',  ( 6.000000000291855429, 2.999999999003851503, -45.00000000000000000 ) ) ;
#7368=EDGE_LOOP ( 'NONE', ( #20781, #8993, #3181, #13708, #20044 ) ) ;
#7377=CARTESIAN_POINT ( 'NONE',  ( 30.00000000029184832, -9.961476088449217059E-10, -3.449999999999999289 ) ) ;
#7386=CARTESIAN_POINT ( 'NONE',  ( 27.94974746859769255, 27.94974746730969528, -15.99999999999999289 ) ) ;
#7396=ORIENTED_EDGE ( 'NONE', *, *, #21338, .F. ) ;
#7399=ORIENTED_EDGE ( 'NONE', *, *, #12376, .T. ) ;
#7408=DIRECTION ( 'NONE',  ( 1.000000000000000000, 0.000000000000000000, 0.000000000000000000 ) ) ;
#7411=DIRECTION ( 'NONE',  ( -0.000000000000000000, -0.000000000000000000, -1.000000000000000000 ) ) ;
#7413=DIRECTION ( 'NONE',  ( 0.7071067811865475727, 0.7071067811865475727, 0.000000000000000000 ) ) ;
#7423=ORIENTED_EDGE ( 'NONE', *, *, #12128, .F. ) ;
#7434=DIRECTION ( 'NONE',  ( 0.000000000000000000, 0.000000000000000000, 1.000000000000000000 ) ) ;
#7449=FACE_OUTER_BOUND ( 'NONE', #9790, .T. ) ;
#7466=AXIS2_PLACEMENT_3D ( 'NONE', #3472, #19822, #19354 ) ;
#7477=ORIENTED_EDGE ( 'NONE', *, *, #21338, .T. ) ;
#7481=ORIENTED_EDGE ( 'NONE', *, *, #5616, .T. ) ;
#7494=DIRECTION ( 'NONE',  ( -0.000000000000000000, -0.000000000000000000, 1.000000000000000000 ) ) ;
#7506=AXIS2_PLACEMENT_3D ( 'NONE', #15836, #17974, #1842 ) ;
#7507=CARTESIAN_POINT ( 'NONE',  ( 2.918498775983380256E-10, -9.961476088449217059E-10, -45.00000000000000000 ) ) ;
#7509=ORIENTED_EDGE ( 'NONE', *, *, #2195, .F. ) ;
#7510=DIRECTION ( 'NONE',  ( 0.000000000000000000, 1.000000000000000000, 0.000000000000000000 ) ) ;
#7512=ADVANCED_FACE ( 'NONE', ( #15014, #6085, #13031 ), #334, .T. ) ;
#7532=LINE ( 'NONE', #5771, #21657 ) ;
#7537=B_SPLINE_CURVE_WITH_KNOTS ( 'NONE', 3,
 ( #23140, #14187, #1824, #10302, #17952, #5366, #5255, #1376, #13942, #12525, #16047, #17472, #23259, #8542, #15702, #6774, #5002, #19360 ),
 .UNSPECIFIED., .F., .F.,
 ( 4, 2, 2, 2, 2, 2, 2, 2, 4 ),
 ( 0.000000000000000000, 0.0005979442104825548809, 0.001195888420965109762, 0.001793832631447664534, 0.002391776841930219524, 0.002989721052412774513, 0.003587665262895329069, 0.004185609473377884492, 0.004783553683860439047 ),
 .UNSPECIFIED. ) ;
#7538=ORIENTED_EDGE ( 'NONE', *, *, #22942, .T. ) ;
#7543=DIRECTION ( 'NONE',  ( 0.000000000000000000, 1.000000000000000000, 0.000000000000000000 ) ) ;
#7559=CARTESIAN_POINT ( 'NONE',  ( 6.000000000291855429, -0.5000000009961480529, -8.549999999999998934 ) ) ;
#7560=PLANE ( 'NONE',  #692 ) ;
#7575=EDGE_CURVE ( 'NONE', #888, #8962, #20999, .T. ) ;
#7576=CARTESIAN_POINT ( 'NONE',  ( 2.918498775983380256E-10, 6.999999999003851947, -15.99999999999999289 ) ) ;
#7588=LINE ( 'NONE', #1933, #23185 ) ;
#7593=ORIENTED_EDGE ( 'NONE', *, *, #325, .F. ) ;
#7623=CARTESIAN_POINT ( 'NONE',  ( -6.649675532656710075, 36.01889503913412227, -27.42797899728712352 ) ) ;
#7624=DIRECTION ( 'NONE',  ( 0.000000000000000000, 0.000000000000000000, 1.000000000000000000 ) ) ;
#7638=DIRECTION ( 'NONE',  ( 1.000000000000000000, 0.000000000000000000, 0.000000000000000000 ) ) ;
#7643=EDGE_CURVE ( 'NONE', #22557, #145, #3021, .T. ) ;
#7645=FACE_BOUND ( 'NONE', #12325, .T. ) ;
#7654=EDGE_CURVE ( 'NONE', #4543, #10008, #4667, .T. ) ;
#7656=ADVANCED_FACE ( 'NONE', ( #18909 ), #13376, .T. ) ;
#7659=CARTESIAN_POINT ( 'NONE',  ( 2.918498775983380256E-10, 2.999999999003851503, -45.00000000000000000 ) ) ;
#7661=ORIENTED_EDGE ( 'NONE', *, *, #2788, .F. ) ;
#7681=TOROIDAL_SURFACE ( 'NONE', #10310, 6.500000000000000888, 0.5000000000000000000 ) ;
#7691=EDGE_LOOP ( 'NONE', ( #13301, #13954 ) ) ;
#7693=CARTESIAN_POINT ( 'NONE',  ( 0.4500000002918510544, 42.99999999900385461, -29.00000000000000355 ) ) ;
#7724=CARTESIAN_POINT ( 'NONE',  ( -6.999999999708142795, 38.99999999900385461, -26.00000000000000000 ) ) ;
#7732=DIRECTION ( 'NONE',  ( -0.000000000000000000, -0.000000000000000000, 1.000000000000000000 ) ) ;
#7733=CARTESIAN_POINT ( 'NONE',  ( -6.962001439796708269, 35.99999999900384751, -26.47597002942762145 ) ) ;
#7761=EDGE_CURVE ( 'NONE', #2264, #12125, #17958, .T. ) ;
#7770=DIRECTION ( 'NONE',  ( 0.000000000000000000, 1.000000000000000000, 0.000000000000000000 ) ) ;
#7774=DIRECTION ( 'NONE',  ( 0.000000000000000000, 0.000000000000000000, 1.000000000000000000 ) ) ;
#7787=CARTESIAN_POINT ( 'NONE',  ( -3.999999999708153453, 42.99999999900385461, -15.99999999999999289 ) ) ;
#7796=ORIENTED_EDGE ( 'NONE', *, *, #9880, .T. ) ;
#7806=DIRECTION ( 'NONE',  ( 1.000000000000000000, 0.000000000000000000, 0.000000000000000000 ) ) ;
#7816=EDGE_CURVE ( 'NONE', #22431, #22269, #12646, .T. ) ;
#7836=( GEOMETRIC_REPRESENTATION_CONTEXT ( 3 ) GLOBAL_UNCERTAINTY_ASSIGNED_CONTEXT ( ( #11207 ) ) GLOBAL_UNIT_ASSIGNED_CONTEXT ( ( #17292, #19413, #17774 ) ) REPRESENTATION_CONTEXT ( 'NONE', 'WORKASPACE' ) );
#7844=DIRECTION ( 'NONE',  ( -0.000000000000000000, 1.000000000000000000, -0.000000000000000000 ) ) ;
#7853=VERTEX_POINT ( 'NONE', #20298 ) ;
#7859=VECTOR ( 'NONE', #14192, 1000.000000000000000 ) ;
#7860=CARTESIAN_POINT ( 'NONE',  ( 36.00000000029184832, 16.99999999900385461, -15.99999999999999289 ) ) ;
#7866=DIRECTION ( 'NONE',  ( 0.000000000000000000, -1.000000000000000000, 0.000000000000000000 ) ) ;
#7889=ORIENTED_EDGE ( 'NONE', *, *, #10538, .F. ) ;
#7896=VECTOR ( 'NONE', #11067, 1000.000000000000000 ) ;
#7898=LINE ( 'NONE', #20140, #14369 ) ;
#7904=ORIENTED_EDGE ( 'NONE', *, *, #21449, .F. ) ;
#7915=CARTESIAN_POINT ( 'NONE',  ( 36.00000000029184832, -9.961476088449217059E-10, 0.000000000000000000 ) ) ;
#7926=LINE ( 'NONE', #13460, #23081 ) ;
#7936=ADVANCED_FACE ( 'NONE', ( #9469 ), #2057, .F. ) ;
#7937=ORIENTED_EDGE ( 'NONE', *, *, #19146, .T. ) ;
#7942=VERTEX_POINT ( 'NONE', #7367 ) ;
#7947=AXIS2_PLACEMENT_3D ( 'NONE', #17055, #9659, #731 ) ;
#7954=DIRECTION ( 'NONE',  ( -1.000000000000000000, 0.000000000000000000, 0.000000000000000000 ) ) ;
#7957=CARTESIAN_POINT ( 'NONE',  ( 7.949747468597695210, 47.94974746730969173, -29.00000000000000355 ) ) ;
#7958=LINE ( 'NONE', #18904, #11140 ) ;
#7978=DIRECTION ( 'NONE',  ( 0.000000000000000000, 0.000000000000000000, 1.000000000000000000 ) ) ;
#7980=CARTESIAN_POINT ( 'NONE',  ( -4.720100440590782931, 36.44386358679986415, -19.00000000000000355 ) ) ;
#7982=LINE ( 'NONE', #703, #10805 ) ;
#7985=AXIS2_PLACEMENT_3D ( 'NONE', #13962, #12311, #9028 ) ;
#8041=DIRECTION ( 'NONE',  ( 0.000000000000000000, 0.000000000000000000, -1.000000000000000000 ) ) ;
#8045=DIRECTION ( 'NONE',  ( -0.000000000000000000, -0.000000000000000000, 1.000000000000000000 ) ) ;
#8056=ORIENTED_EDGE ( 'NONE', *, *, #20454, .F. ) ;
#8058=ORIENTED_EDGE ( 'NONE', *, *, #2173, .T. ) ;
#8095=CARTESIAN_POINT ( 'NONE',  ( 29.00000000029184832, 16.99999999900385461, -26.00000000000000000 ) ) ;
#8097=EDGE_CURVE ( 'NONE', #178, #10008, #14749, .T. ) ;
#8100=CARTESIAN_POINT ( 'NONE',  ( -4.550510256924973795, 35.99999999900384751, -19.00000000000000000 ) ) ;
#8125=DIRECTION ( 'NONE',  ( -0.000000000000000000, -0.000000000000000000, -1.000000000000000000 ) ) ;
#8144=ORIENTED_EDGE ( 'NONE', *, *, #21222, .T. ) ;
#8151=VERTEX_POINT ( 'NONE', #22094 ) ;
#8162=VECTOR ( 'NONE', #4584, 1000.000000000000000 ) ;
#8172=CIRCLE ( 'NONE', #21333, 6.000000000000000000 ) ;
#8180=EDGE_CURVE ( 'NONE', #2292, #4761, #18998, .T. ) ;
#8187=DIRECTION ( 'NONE',  ( 0.000000000000000000, 0.000000000000000000, 1.000000000000000000 ) ) ;
#8190=CARTESIAN_POINT ( 'NONE',  ( 3.000000000291852764, 42.99999999900385461, -19.00000000000000355 ) ) ;
#8199=CARTESIAN_POINT ( 'NONE',  ( 3.000000000291852764, 42.99999999900385461, -15.99999999999999289 ) ) ;
#8203=LINE ( 'NONE', #19026, #11172 ) ;
#8213=ORIENTED_EDGE ( 'NONE', *, *, #6505, .T. ) ;
#8215=CARTESIAN_POINT ( 'NONE',  ( 2.918498775983380256E-10, 2.999999999003851503, 0.000000000000000000 ) ) ;
#8216=DIRECTION ( 'NONE',  ( -0.000000000000000000, -0.000000000000000000, 1.000000000000000000 ) ) ;
#8226=DIRECTION ( 'NONE',  ( -0.000000000000000000, 1.000000000000000000, -0.000000000000000000 ) ) ;
#8252=DIRECTION ( 'NONE',  ( 0.000000000000000000, -1.000000000000000000, 0.000000000000000000 ) ) ;
#8262=EDGE_LOOP ( 'NONE', ( #4952, #4607, #21324, #3917, #17788, #4249, #4394 ) ) ;
#8273=DIRECTION ( 'NONE',  ( 0.000000000000000000, 0.000000000000000000, -1.000000000000000000 ) ) ;
#8275=DIRECTION ( 'NONE',  ( 0.000000000000000000, 0.000000000000000000, 1.000000000000000000 ) ) ;
#8282=CARTESIAN_POINT ( 'NONE',  ( 36.00000000029184832, 5.999999999003851059, -12.99999999999999822 ) ) ;
#8287=CYLINDRICAL_SURFACE ( 'NONE', #20965, 6.999999999999999112 ) ;
#8300=DIRECTION ( 'NONE',  ( 0.000000000000000000, 1.000000000000000000, 0.000000000000000000 ) ) ;
#8307=CIRCLE ( 'NONE', #6056, 2.549999999999996714 ) ;
#8310=CARTESIAN_POINT ( 'NONE',  ( 36.00000000029184832, 49.99999999900385461, -28.99999999999999645 ) ) ;
#8315=CARTESIAN_POINT ( 'NONE',  ( 2.918498775983380256E-10, 2.999999999003851503, 0.000000000000000000 ) ) ;
#8327=CARTESIAN_POINT ( 'NONE',  ( 2.918498775983380256E-10, 2.999999999003851503, -45.00000000000000000 ) ) ;
#8347=DIRECTION ( 'NONE',  ( 1.000000000000000000, 0.000000000000000000, 0.000000000000000000 ) ) ;
#8379=VERTEX_POINT ( 'NONE', #15605 ) ;
#8391=DIRECTION ( 'NONE',  ( 1.000000000000000000, 0.000000000000000000, 0.000000000000000000 ) ) ;
#8413=AXIS2_PLACEMENT_3D ( 'NONE', #11165, #464, #7638 ) ;
#8414=ORIENTED_EDGE ( 'NONE', *, *, #5967, .T. ) ;
#8427=AXIS2_PLACEMENT_3D ( 'NONE', #16819, #3815, #18189 ) ;
#8432=CARTESIAN_POINT ( 'NONE',  ( -6.961281259571849844, 35.99999999900387593, -26.48045177140990702 ) ) ;
#8440=DIRECTION ( 'NONE',  ( 0.000000000000000000, -1.000000000000000000, 0.000000000000000000 ) ) ;
#8445=AXIS2_PLACEMENT_3D ( 'NONE', #4233, #22017, #2131 ) ;
#8458=CARTESIAN_POINT ( 'NONE',  ( -3.499999999708153453, 38.99999999900385461, -18.50000000000000355 ) ) ;
#8465=ADVANCED_FACE ( 'NONE', ( #12863 ), #22035, .F. ) ;
#8466=ORIENTED_EDGE ( 'NONE', *, *, #9090, .T. ) ;
#8469=VERTEX_POINT ( 'NONE', #7693 ) ;
#8470=ORIENTED_EDGE ( 'NONE', *, *, #13317, .T. ) ;
#8486=DIRECTION ( 'NONE',  ( -0.000000000000000000, -0.000000000000000000, 1.000000000000000000 ) ) ;
#8488=ORIENTED_EDGE ( 'NONE', *, *, #21771, .T. ) ;
#8503=DIRECTION ( 'NONE',  ( 0.000000000000000000, 0.000000000000000000, 1.000000000000000000 ) ) ;
#8509=DIRECTION ( 'NONE',  ( 0.000000000000000000, 1.000000000000000000, 0.000000000000000000 ) ) ;
#8511=AXIS2_PLACEMENT_3D ( 'NONE', #17706, #15704, #3140 ) ;
#8513=CARTESIAN_POINT ( 'NONE',  ( 29.00000000029184832, 16.99999999900385461, -26.00000000000000000 ) ) ;
#8516=ORIENTED_EDGE ( 'NONE', *, *, #17784, .F. ) ;
#8519=ORIENTED_EDGE ( 'NONE', *, *, #16903, .F. ) ;
#8542=CARTESIAN_POINT ( 'NONE',  ( -6.839530184912448796, 13.99859551563898563, -18.01161035304105695 ) ) ;
#8557=EDGE_LOOP ( 'NONE', ( #9104, #18246, #7034, #12126 ) ) ;
#8570=CARTESIAN_POINT ( 'NONE',  ( 6.000000000291855429, -9.961476088449217059E-10, 0.000000000000000000 ) ) ;
#8578=CARTESIAN_POINT ( 'NONE',  ( 5.550000000291854363, 42.99999999900385461, -19.00000000000000355 ) ) ;
#8585=EDGE_CURVE ( 'NONE', #6752, #8151, #750, .T. ) ;
#8586=VERTEX_POINT ( 'NONE', #2854 ) ;
#8600=SHAPE_REPRESENTATION_RELATIONSHIP ( 'NONE' , 'NONE' ,  #10586, #18435 ) ;
#8602=ADVANCED_FACE ( 'NONE', ( #10031 ), #13448, .F. ) ;
#8609=ORIENTED_EDGE ( 'NONE', *, *, #12894, .T. ) ;
#8612=DIRECTION ( 'NONE',  ( 0.000000000000000000, -1.000000000000000000, 0.000000000000000000 ) ) ;
#8619=DIRECTION ( 'NONE',  ( -1.000000000000000000, 0.000000000000000000, 0.000000000000000000 ) ) ;
#8628=DIRECTION ( 'NONE',  ( 1.000000000000000000, 0.000000000000000000, 0.000000000000000000 ) ) ;
#8632=ORIENTED_EDGE ( 'NONE', *, *, #17731, .T. ) ;
#8642=DIRECTION ( 'NONE',  ( -0.000000000000000000, -0.000000000000000000, 1.000000000000000000 ) ) ;
#8644=ORIENTED_EDGE ( 'NONE', *, *, #6485, .F. ) ;
#8647=CARTESIAN_POINT ( 'NONE',  ( 36.00000000029184832, 16.99999999900385461, -19.49999999999998934 ) ) ;
#8651=FACE_OUTER_BOUND ( 'NONE', #5700, .T. ) ;
#8658=VERTEX_POINT ( 'NONE', #13680 ) ;
#8664=ORIENTED_EDGE ( 'NONE', *, *, #13029, .T. ) ;
#8668=EDGE_CURVE ( 'NONE', #14653, #19191, #6273, .T. ) ;
#8672=AXIS2_PLACEMENT_3D ( 'NONE', #9409, #11163, #19989 ) ;
#8685=FACE_OUTER_BOUND ( 'NONE', #11057, .T. ) ;
#8687=DIRECTION ( 'NONE',  ( 0.000000000000000000, 0.000000000000000000, -1.000000000000000000 ) ) ;
#8691=AXIS2_PLACEMENT_3D ( 'NONE', #2075, #10785, #23162 ) ;
#8704=CARTESIAN_POINT ( 'NONE',  ( 27.94974746859769255, 27.94974746730969528, -26.50000000000000000 ) ) ;
#8705=AXIS2_PLACEMENT_3D ( 'NONE', #19472, #497, #16361 ) ;
#8709=LINE ( 'NONE', #21306, #6527 ) ;
#8721=ORIENTED_EDGE ( 'NONE', *, *, #15256, .F. ) ;
#8722=VECTOR ( 'NONE', #6617, 1000.000000000000000 ) ;
#8736=FACE_OUTER_BOUND ( 'NONE', #19310, .T. ) ;
#8745=DIRECTION ( 'NONE',  ( 1.000000000000000000, 0.000000000000000000, 0.000000000000000000 ) ) ;
#8750=ORIENTED_EDGE ( 'NONE', *, *, #2773, .T. ) ;
#8753=VERTEX_POINT ( 'NONE', #7204 ) ;
#8757=CIRCLE ( 'NONE', #4615, 5.999999999999998224 ) ;
#8759=EDGE_LOOP ( 'NONE', ( #12057, #7796, #9685, #6606, #21468, #17605 ) ) ;
#8760=LINE ( 'NONE', #17824, #15176 ) ;
#8770=CARTESIAN_POINT ( 'NONE',  ( -6.959810536856680940, 36.00015702695179698, -26.48940942388196618 ) ) ;
#8781=CIRCLE ( 'NONE', #7947, 2.999999999999999112 ) ;
#8792=VECTOR ( 'NONE', #10076, 1000.000000000000000 ) ;
#8799=CARTESIAN_POINT ( 'NONE',  ( 2.918498775983380256E-10, 2.999999999003851503, 0.000000000000000000 ) ) ;
#8814=ORIENTED_EDGE ( 'NONE', *, *, #16257, .T. ) ;
#8818=EDGE_CURVE ( 'NONE', #14256, #22384, #6639, .T. ) ;
#8820=ORIENTED_EDGE ( 'NONE', *, *, #3459, .F. ) ;
#8826=ORIENTED_EDGE ( 'NONE', *, *, #14274, .T. ) ;
#8840=FILL_AREA_STYLE_COLOUR ( '', #23256 ) ;
#8853=CARTESIAN_POINT ( 'NONE',  ( -6.999999999708156118, 6.999999999003851947, -29.00000000000000355 ) ) ;
#8854=DIRECTION ( 'NONE',  ( 0.000000000000000000, 0.000000000000000000, -1.000000000000000000 ) ) ;
#8873=ORIENTED_EDGE ( 'NONE', *, *, #32, .T. ) ;
#8885=FACE_OUTER_BOUND ( 'NONE', #12447, .T. ) ;
#8886=CARTESIAN_POINT ( 'NONE',  ( -6.958637146882876934, 36.00028510068597143, -26.49646658807206379 ) ) ;
#8932=CARTESIAN_POINT ( 'NONE',  ( -6.975867733732471265, 36.00005661733526807, -26.49364064955104681 ) ) ;
#8957=AXIS2_PLACEMENT_3D ( 'NONE', #11746, #4697, #6695 ) ;
#8962=VERTEX_POINT ( 'NONE', #11290 ) ;
#8964=VERTEX_POINT ( 'NONE', #4000 ) ;
#8973=DIRECTION ( 'NONE',  ( 0.000000000000000000, 0.000000000000000000, -1.000000000000000000 ) ) ;
#8982=DIRECTION ( 'NONE',  ( -1.858632295689435609E-16, -1.000000000000000000, 2.999267978177796234E-32 ) ) ;
#8991=VERTEX_POINT ( 'NONE', #2828 ) ;
#8993=ORIENTED_EDGE ( 'NONE', *, *, #13223, .T. ) ;
#8999=VERTEX_POINT ( 'NONE', #18821 ) ;
#9015=VECTOR ( 'NONE', #13069, 1000.000000000000000 ) ;
#9024=CYLINDRICAL_SURFACE ( 'NONE', #20817, 7.000000000000006217 ) ;
#9028=DIRECTION ( 'NONE',  ( 0.000000000000000000, 0.000000000000000000, 1.000000000000000000 ) ) ;
#9036=DIRECTION ( 'NONE',  ( -1.000000000000000000, 0.000000000000000000, 0.000000000000000000 ) ) ;
#9043=CARTESIAN_POINT ( 'NONE',  ( -5.403531933167076140, 36.45753077221091587, -28.65347769269738976 ) ) ;
#9051=DIRECTION ( 'NONE',  ( 0.000000000000000000, 0.000000000000000000, 1.000000000000000000 ) ) ;
#9060=CARTESIAN_POINT ( 'NONE',  ( -3.499999999708153453, 35.49999999900384751, -19.50000000000000355 ) ) ;
#9080=CARTESIAN_POINT ( 'NONE',  ( 3.000000000291852764, 42.99999999900385461, -26.50000000000000000 ) ) ;
#9090=EDGE_CURVE ( 'NONE', #12443, #22242, #13299, .T. ) ;
#9093=VERTEX_POINT ( 'NONE', #4706 ) ;
#9104=ORIENTED_EDGE ( 'NONE', *, *, #14098, .F. ) ;
#9106=ADVANCED_FACE ( 'NONE', ( #9768 ), #22364, .F. ) ;
#9113=DIRECTION ( 'NONE',  ( 0.000000000000000000, 0.000000000000000000, 1.000000000000000000 ) ) ;
#9127=DIRECTION ( 'NONE',  ( 0.000000000000000000, 0.000000000000000000, -1.000000000000000000 ) ) ;
#9136=ORIENTED_EDGE ( 'NONE', *, *, #6066, .T. ) ;
#9151=AXIS2_PLACEMENT_3D ( 'NONE', #1782, #7101, #7207 ) ;
#9160=VERTEX_POINT ( 'NONE', #19521 ) ;
#9162=CIRCLE ( 'NONE', #13295, 3.000000000000000000 ) ;
#9164=AXIS2_PLACEMENT_3D ( 'NONE', #2222, #20107, #7408 ) ;
#9170=DIRECTION ( 'NONE',  ( -0.000000000000000000, 1.000000000000000000, -0.000000000000000000 ) ) ;
#9198=CARTESIAN_POINT ( 'NONE',  ( -4.550510256924974684, 35.99999999900384751, -25.50000000000000000 ) ) ;
#9201=LINE ( 'NONE', #5093, #6177 ) ;
#9211=CARTESIAN_POINT ( 'NONE',  ( -4.990285246490005377, 35.99999999900386172, -19.46466550946063023 ) ) ;
#9215=ORIENTED_EDGE ( 'NONE', *, *, #8668, .T. ) ;
#9223=ORIENTED_EDGE ( 'NONE', *, *, #21666, .T. ) ;
#9233=LINE ( 'NONE', #3931, #6704 ) ;
#9234=DIRECTION ( 'NONE',  ( -0.000000000000000000, -1.000000000000000000, -0.000000000000000000 ) ) ;
#9236=DIRECTION ( 'NONE',  ( -0.000000000000000000, 1.000000000000000000, 0.000000000000000000 ) ) ;
#9278=CARTESIAN_POINT ( 'NONE',  ( -4.950765356264097861, 36.36782871084110980, -18.97560888259267387 ) ) ;
#9281=CIRCLE ( 'NONE', #15276, 2.550000000000003819 ) ;
#9287=CIRCLE ( 'NONE', #2136, 2.550000000000000266 ) ;
#9288=FACE_OUTER_BOUND ( 'NONE', #12185, .T. ) ;
#9289=DIRECTION ( 'NONE',  ( 0.000000000000000000, -1.000000000000000000, 0.000000000000000000 ) ) ;
#9292=CARTESIAN_POINT ( 'NONE',  ( 30.00000000029184832, -9.961476088449217059E-10, -41.54999999999999716 ) ) ;
#9305=ORIENTED_EDGE ( 'NONE', *, *, #20882, .F. ) ;
#9315=CARTESIAN_POINT ( 'NONE',  ( -5.403531933167068146, 36.45753077221091587, -16.34652230730261380 ) ) ;
#9322=CARTESIAN_POINT ( 'NONE',  ( 30.00000000029184832, 2.999999999003851503, -39.00000000000000000 ) ) ;
#9331=ORIENTED_EDGE ( 'NONE', *, *, #17269, .T. ) ;
#9356=AXIS2_PLACEMENT_3D ( 'NONE', #13537, #8125, #20951 ) ;
#9358=ORIENTED_EDGE ( 'NONE', *, *, #348, .T. ) ;
#9369=ORIENTED_EDGE ( 'NONE', *, *, #6231, .T. ) ;
#9382=DIRECTION ( 'NONE',  ( -0.000000000000000000, 1.000000000000000000, 0.000000000000000000 ) ) ;
#9398=CARTESIAN_POINT ( 'NONE',  ( -4.751720029897056996, 36.43339712399806274, -19.00000000000001066 ) ) ;
#9405=EDGE_CURVE ( 'NONE', #4871, #8586, #3236, .T. ) ;
#9409=CARTESIAN_POINT ( 'NONE',  ( 35.50000000029184832, 2.999999999003851503, -26.50000000000000000 ) ) ;
#9413=DIRECTION ( 'NONE',  ( -1.000000000000000000, 0.000000000000000000, 0.000000000000000000 ) ) ;
#9415=EDGE_CURVE ( 'NONE', #343, #3554, #21865, .T. ) ;
#9438=CARTESIAN_POINT ( 'NONE',  ( -3.999999999708153453, 38.99999999900385461, -26.50000000000000000 ) ) ;
#9462=DIRECTION ( 'NONE',  ( 0.000000000000000000, 0.000000000000000000, -1.000000000000000000 ) ) ;
#9469=FACE_OUTER_BOUND ( 'NONE', #16116, .T. ) ;
#9476=VECTOR ( 'NONE', #15954, 1000.000000000000000 ) ;
#9483=VECTOR ( 'NONE', #3569, 1000.000000000000000 ) ;
#9511=AXIS2_PLACEMENT_3D ( 'NONE', #2974, #8273, #9920 ) ;
#9514=LINE ( 'NONE', #11041, #21931 ) ;
#9525=DIRECTION ( 'NONE',  ( 1.858632295689435609E-16, 1.000000000000000000, -0.000000000000000000 ) ) ;
#9528=CIRCLE ( 'NONE', #2384, 6.000000000000000000 ) ;
#9530=TOROIDAL_SURFACE ( 'NONE', #5795, 1.000000000000000000, 0.5000000000000000000 ) ;
#9532=AXIS2_PLACEMENT_3D ( 'NONE', #12131, #19321, #3215 ) ;
#9552=PLANE ( 'NONE',  #8705 ) ;
#9567=ORIENTED_EDGE ( 'NONE', *, *, #1648, .F. ) ;
#9576=FILL_AREA_STYLE_COLOUR ( '', #18584 ) ;
#9604=LINE ( 'NONE', #4070, #459 ) ;
#9611=CYLINDRICAL_SURFACE ( 'NONE', #344, 2.549999999999998934 ) ;
#9621=ORIENTED_EDGE ( 'NONE', *, *, #18243, .T. ) ;
#9626=AXIS2_PLACEMENT_3D ( 'NONE', #10531, #10071, #17233 ) ;
#9646=CIRCLE ( 'NONE', #13041, 0.4999999999999982236 ) ;
#9656=CARTESIAN_POINT ( 'NONE',  ( -5.122455540400322249, 36.64919863988808402, -16.21011172720200477 ) ) ;
#9659=DIRECTION ( 'NONE',  ( -1.000000000000000000, 0.000000000000000000, 0.000000000000000000 ) ) ;
#9674=ORIENTED_EDGE ( 'NONE', *, *, #13156, .F. ) ;
#9685=ORIENTED_EDGE ( 'NONE', *, *, #20454, .T. ) ;
#9694=AXIS2_PLACEMENT_3D ( 'NONE', #10271, #22869, #4973 ) ;
#9698=AXIS2_PLACEMENT_3D ( 'NONE', #1020, #22422, #20670 ) ;
#9713=AXIS2_PLACEMENT_3D ( 'NONE', #10926, #14127, #134 ) ;
#9724=CYLINDRICAL_SURFACE ( 'NONE', #6863, 2.550000000000003819 ) ;
#9732=CARTESIAN_POINT ( 'NONE',  ( -3.999999999708153453, 42.99999999900385461, -15.50000000000000000 ) ) ;
#9747=DIRECTION ( 'NONE',  ( 1.000000000000000000, 0.000000000000000000, 0.000000000000000000 ) ) ;
#9753=CARTESIAN_POINT ( 'NONE',  ( -6.605954977391715666, 35.99999999900384751, -18.74919553276986761 ) ) ;
#9768=FACE_OUTER_BOUND ( 'NONE', #10189, .T. ) ;
#9774=CARTESIAN_POINT ( 'NONE',  ( -3.999999999708153453, 35.49999999900384751, -22.50000000000000000 ) ) ;
#9775=CYLINDRICAL_SURFACE ( 'NONE', #12603, 0.5000000000000004441 ) ;
#9776=FACE_OUTER_BOUND ( 'NONE', #6157, .T. ) ;
#9778=CARTESIAN_POINT ( 'NONE',  ( 31.55000000029185259, 16.99999999900385461, -26.00000000000000000 ) ) ;
#9785=VERTEX_POINT ( 'NONE', #19843 ) ;
#9787=ORIENTED_EDGE ( 'NONE', *, *, #17419, .T. ) ;
#9790=EDGE_LOOP ( 'NONE', ( #2940, #10253, #1914, #3882 ) ) ;
#9800=( NAMED_UNIT ( * ) SI_UNIT ( $, .STERADIAN. ) SOLID_ANGLE_UNIT ( ) );
#9805=DIRECTION ( 'NONE',  ( 0.000000000000000000, 1.000000000000000000, 0.000000000000000000 ) ) ;
#9817=ORIENTED_EDGE ( 'NONE', *, *, #4461, .F. ) ;
#9820=ORIENTED_EDGE ( 'NONE', *, *, #6538, .F. ) ;
#9854=ORIENTED_EDGE ( 'NONE', *, *, #6241, .F. ) ;
#9856=DIRECTION ( 'NONE',  ( 0.000000000000000000, 0.000000000000000000, 1.000000000000000000 ) ) ;
#9863=CARTESIAN_POINT ( 'NONE',  ( -5.471017171497492448, 36.21317998573887564, -18.88264757256944293 ) ) ;
#9880=EDGE_CURVE ( 'NONE', #145, #19937, #16754, .T. ) ;
#9881=VECTOR ( 'NONE', #15523, 1000.000000000000000 ) ;
#9886=ORIENTED_EDGE ( 'NONE', *, *, #7761, .T. ) ;
#9892=CYLINDRICAL_SURFACE ( 'NONE', #10550, 2.550000000000003819 ) ;
#9893=LINE ( 'NONE', #1082, #9881 ) ;
#9899=DIRECTION ( 'NONE',  ( -0.000000000000000000, -0.000000000000000000, 1.000000000000000000 ) ) ;
#9905=AXIS2_PLACEMENT_3D ( 'NONE', #15048, #2356, #20487 ) ;
#9909=EDGE_LOOP ( 'NONE', ( #4429, #4811, #1911, #2058, #18850, #4841, #20535 ) ) ;
#9910=EDGE_CURVE ( 'NONE', #16865, #16772, #10061, .T. ) ;
#9920=DIRECTION ( 'NONE',  ( 1.000000000000000000, 0.000000000000000000, 0.000000000000000000 ) ) ;
#9924=DIRECTION ( 'NONE',  ( 0.000000000000000000, -1.000000000000000000, 0.000000000000000000 ) ) ;
#9937=CARTESIAN_POINT ( 'NONE',  ( -5.945013150601167418, 13.92153864138982300, -28.29267684501254010 ) ) ;
#9944=EDGE_LOOP ( 'NONE', ( #6237, #11428 ) ) ;
#9956=FACE_OUTER_BOUND ( 'NONE', #176, .T. ) ;
#9962=EDGE_CURVE ( 'NONE', #11848, #12207, #4760, .T. ) ;
#9965=DIRECTION ( 'NONE',  ( -1.613696256722611405E-16, 0.000000000000000000, 1.000000000000000000 ) ) ;
#9967=DIRECTION ( 'NONE',  ( 0.000000000000000000, -1.000000000000000000, 0.000000000000000000 ) ) ;
#9973=ADVANCED_FACE ( 'NONE', ( #20544 ), #15223, .F. ) ;
#9981=ORIENTED_EDGE ( 'NONE', *, *, #20987, .F. ) ;
#9987=DIRECTION ( 'NONE',  ( -0.7071067811865492381, -0.7071067811865457964, 0.000000000000000000 ) ) ;
#10008=VERTEX_POINT ( 'NONE', #6648 ) ;
#10031=FACE_OUTER_BOUND ( 'NONE', #17420, .T. ) ;
#10032=CARTESIAN_POINT ( 'NONE',  ( 36.00000000029184832, 2.999999999003851503, -45.00000000000000000 ) ) ;
#10033=DIRECTION ( 'NONE',  ( -1.000000000000000000, 0.000000000000000000, 0.000000000000000000 ) ) ;
#10044=CARTESIAN_POINT ( 'NONE',  ( 2.918498775983380256E-10, 2.999999999003851503, -5.999999999999998224 ) ) ;
#10055=ORIENTED_EDGE ( 'NONE', *, *, #7654, .F. ) ;
#10058=ORIENTED_EDGE ( 'NONE', *, *, #1681, .F. ) ;
#10061=LINE ( 'NONE', #11824, #20397 ) ;
#10071=DIRECTION ( 'NONE',  ( -1.613696256722611405E-16, 0.000000000000000000, -1.000000000000000000 ) ) ;
#10076=DIRECTION ( 'NONE',  ( 0.000000000000000000, 1.000000000000000000, -0.000000000000000000 ) ) ;
#10078=DIRECTION ( 'NONE',  ( 1.000000000000000000, 0.000000000000000000, 0.000000000000000000 ) ) ;
#10095=DIRECTION ( 'NONE',  ( 1.000000000000000000, -0.000000000000000000, 0.000000000000000000 ) ) ;
#10099=CARTESIAN_POINT ( 'NONE',  ( -5.311293330718551253, 35.99999999900384751, -19.06129441391418666 ) ) ;
#10100=CARTESIAN_POINT ( 'NONE',  ( -3.499999999708153453, 13.99999999900385106, -19.00000000000000355 ) ) ;
#10108=DIRECTION ( 'NONE',  ( 0.000000000000000000, 0.000000000000000000, 1.000000000000000000 ) ) ;
#10116=VERTEX_POINT ( 'NONE', #21247 ) ;
#10124=DIRECTION ( 'NONE',  ( -1.000000000000000000, 0.000000000000000000, 0.000000000000000000 ) ) ;
#10134=LINE ( 'NONE', #15298, #16036 ) ;
#10145=ORIENTED_EDGE ( 'NONE', *, *, #21054, .F. ) ;
#10161=CARTESIAN_POINT ( 'NONE',  ( -6.979783269036460069, 14.00008466144083030, -26.40130824240443275 ) ) ;
#10166=ORIENTED_EDGE ( 'NONE', *, *, #7816, .T. ) ;
#10178=AXIS2_PLACEMENT_3D ( 'NONE', #21069, #19063, #23189 ) ;
#10189=EDGE_LOOP ( 'NONE', ( #21809, #4896, #12589 ) ) ;
#10210=FACE_BOUND ( 'NONE', #1916, .T. ) ;
#10219=AXIS2_PLACEMENT_3D ( 'NONE', #17581, #8187, #1017 ) ;
#10231=CARTESIAN_POINT ( 'NONE',  ( 2.918498775983380256E-10, 2.999999999003851503, -12.99999999999999822 ) ) ;
#10238=AXIS2_PLACEMENT_3D ( 'NONE', #14412, #12277, #9113 ) ;
#10251=ORIENTED_EDGE ( 'NONE', *, *, #11153, .T. ) ;
#10253=ORIENTED_EDGE ( 'NONE', *, *, #21581, .T. ) ;
#10264=DIRECTION ( 'NONE',  ( 0.000000000000000000, -1.000000000000000000, 0.000000000000000000 ) ) ;
#10271=CARTESIAN_POINT ( 'NONE',  ( -3.499999999708153453, 38.99999999900385461, -26.50000000000000000 ) ) ;
#10290=FACE_OUTER_BOUND ( 'NONE', #524, .T. ) ;
#10302=CARTESIAN_POINT ( 'NONE',  ( -4.733938537004360292, 13.62597557122357372, -16.08514644908176905 ) ) ;
#10306=DIRECTION ( 'NONE',  ( 0.000000000000000000, 0.000000000000000000, 1.000000000000000000 ) ) ;
#10310=AXIS2_PLACEMENT_3D ( 'NONE', #9080, #12247, #23106 ) ;
#10356=EDGE_CURVE ( 'NONE', #283, #5825, #20520, .T. ) ;
#10365=VERTEX_POINT ( 'NONE', #22161 ) ;
#10375=CARTESIAN_POINT ( 'NONE',  ( -3.499999999708153453, 35.49999999900384751, -26.00000000000000000 ) ) ;
#10396=VERTEX_POINT ( 'NONE', #4264 ) ;
#10404=EDGE_CURVE ( 'NONE', #12740, #22474, #19643, .T. ) ;
#10425=ORIENTED_EDGE ( 'NONE', *, *, #3651, .F. ) ;
#10431=VECTOR ( 'NONE', #14722, 1000.000000000000000 ) ;
#10450=CARTESIAN_POINT ( 'NONE',  ( -6.999999999708142795, 13.99999999900385106, -19.00000000000000355 ) ) ;
#10452=CARTESIAN_POINT ( 'NONE',  ( 29.00000000029184832, 16.99999999900385461, -26.50000000000000000 ) ) ;
#10460=CARTESIAN_POINT ( 'NONE',  ( -4.896882909240444448, 36.38534960922712713, -26.01795247534147393 ) ) ;
#10467=ORIENTED_EDGE ( 'NONE', *, *, #8097, .F. ) ;
#10469=LINE ( 'NONE', #17637, #736 ) ;
#10478=VECTOR ( 'NONE', #379, 1000.000000000000000 ) ;
#10528=CARTESIAN_POINT ( 'NONE',  ( -6.958039891257955745, 36.00029345514013102, -26.50000000000000000 ) ) ;
#10531=CARTESIAN_POINT ( 'NONE',  ( 36.00000000029184832, 49.99999999900385461, -16.00000000000000000 ) ) ;
#10536=CYLINDRICAL_SURFACE ( 'NONE', #8511, 2.549999999999996714 ) ;
#10538=EDGE_CURVE ( 'NONE', #6361, #8991, #124, .T. ) ;
#10541=CARTESIAN_POINT ( 'NONE',  ( -4.365918574175958078, 13.48846683486500808, -28.98347793635020864 ) ) ;
#10550=AXIS2_PLACEMENT_3D ( 'NONE', #20491, #7770, #16928 ) ;
#10555=LINE ( 'NONE', #8799, #9476 ) ;
#10559=DIRECTION ( 'NONE',  ( -0.000000000000000000, 1.000000000000000000, -0.000000000000000000 ) ) ;
#10570=CARTESIAN_POINT ( 'NONE',  ( -6.979889398518855259, 35.99999999900384751, -26.48728129910209006 ) ) ;
#10578=ORIENTED_EDGE ( 'NONE', *, *, #17415, .T. ) ;
#10586=SHAPE_REPRESENTATION ( 'Base', ( #22115 ), #7836 ) ;
#10591=ORIENTED_EDGE ( 'NONE', *, *, #21353, .F. ) ;
#10592=AXIS2_PLACEMENT_3D ( 'NONE', #1087, #8252, #22373 ) ;
#10596=ORIENTED_EDGE ( 'NONE', *, *, #8585, .F. ) ;
#10602=ORIENTED_EDGE ( 'NONE', *, *, #7246, .F. ) ;
#10614=EDGE_CURVE ( 'NONE', #21236, #13097, #9514, .T. ) ;
#10621=ORIENTED_EDGE ( 'NONE', *, *, #22938, .F. ) ;
#10625=CIRCLE ( 'NONE', #8445, 0.5000000000000004441 ) ;
#10634=ORIENTED_EDGE ( 'NONE', *, *, #2745, .F. ) ;
#10641=FACE_OUTER_BOUND ( 'NONE', #8557, .T. ) ;
#10659=ORIENTED_EDGE ( 'NONE', *, *, #6064, .F. ) ;
#10672=EDGE_CURVE ( 'NONE', #8469, #3083, #2011, .T. ) ;
#10674=CARTESIAN_POINT ( 'NONE',  ( -3.499999999708153453, 42.99999999900385461, -19.00000000000000355 ) ) ;
#10689=CARTESIAN_POINT ( 'NONE',  ( -6.130979318138412459, 35.99999999900384751, -26.13052066537846940 ) ) ;
#10708=DIRECTION ( 'NONE',  ( -0.000000000000000000, 1.000000000000000000, -0.000000000000000000 ) ) ;
#10723=AXIS2_PLACEMENT_3D ( 'NONE', #12907, #16072, #2076 ) ;
#10727=ADVANCED_FACE ( 'NONE', ( #12068 ), #6676, .F. ) ;
#10754=CYLINDRICAL_SURFACE ( 'NONE', #4965, 0.4999999999999982236 ) ;
#10764=DIRECTION ( 'NONE',  ( 1.000000000000000000, 0.000000000000000000, 0.000000000000000000 ) ) ;
#10773=ORIENTED_EDGE ( 'NONE', *, *, #23059, .T. ) ;
#10784=PLANE ( 'NONE',  #7506 ) ;
#10785=DIRECTION ( 'NONE',  ( 0.000000000000000000, -1.000000000000000000, 0.000000000000000000 ) ) ;
#10797=VECTOR ( 'NONE', #8982, 1000.000000000000000 ) ;
#10805=VECTOR ( 'NONE', #7866, 1000.000000000000000 ) ;
#10816=CARTESIAN_POINT ( 'NONE',  ( -3.499999999708153453, 42.99999999900385461, -18.50000000000000355 ) ) ;
#10844=AXIS2_PLACEMENT_3D ( 'NONE', #4083, #7732, #11259 ) ;
#10862=ORIENTED_EDGE ( 'NONE', *, *, #21508, .F. ) ;
#10887=FACE_OUTER_BOUND ( 'NONE', #20113, .T. ) ;
#10897=DIRECTION ( 'NONE',  ( 0.000000000000000000, 0.000000000000000000, -1.000000000000000000 ) ) ;
#10911=CARTESIAN_POINT ( 'NONE',  ( 30.00000000029184832, -9.961476088449217059E-10, -45.00000000000000000 ) ) ;
#10925=EDGE_CURVE ( 'NONE', #10008, #178, #17740, .T. ) ;
#10926=CARTESIAN_POINT ( 'NONE',  ( 3.000000000291852764, 42.99999999900385461, -25.50000000000000355 ) ) ;
#10933=EDGE_CURVE ( 'NONE', #3970, #371, #23024, .T. ) ;
#10956=CARTESIAN_POINT ( 'NONE',  ( -6.219322015043732499, 35.99999999900384040, -18.99225239120474740 ) ) ;
#10960=EDGE_CURVE ( 'NONE', #22262, #12387, #10555, .T. ) ;
#10980=DIRECTION ( 'NONE',  ( 0.7071067811865475727, -0.7071067811865475727, 0.000000000000000000 ) ) ;
#11013=VECTOR ( 'NONE', #15861, 1000.000000000000114 ) ;
#11015=DIRECTION ( 'NONE',  ( 0.000000000000000000, 0.000000000000000000, 1.000000000000000000 ) ) ;
#11033=CARTESIAN_POINT ( 'NONE',  ( -4.499999999708154341, 36.49999999900384751, -19.50000000000000355 ) ) ;
#11034=ORIENTED_EDGE ( 'NONE', *, *, #974, .T. ) ;
#11041=CARTESIAN_POINT ( 'NONE',  ( -3.999999999708153453, 36.49999999900384751, -26.00000000000000000 ) ) ;
#11044=CARTESIAN_POINT ( 'NONE',  ( -6.999999999708156118, 6.999999999003851947, -26.00000000000000000 ) ) ;
#11051=LINE ( 'NONE', #14928, #5592 ) ;
#11057=EDGE_LOOP ( 'NONE', ( #3910, #15603, #8488, #6043 ) ) ;
#11067=DIRECTION ( 'NONE',  ( -0.000000000000000000, 1.000000000000000000, -0.000000000000000000 ) ) ;
#11072=FACE_OUTER_BOUND ( 'NONE', #18906, .T. ) ;
#11083=ORIENTED_EDGE ( 'NONE', *, *, #17731, .F. ) ;
#11088=VERTEX_POINT ( 'NONE', #14892 ) ;
#11115=ORIENTED_EDGE ( 'NONE', *, *, #20303, .T. ) ;
#11117=ADVANCED_FACE ( 'NONE', ( #6547 ), #9724, .F. ) ;
#11119=ORIENTED_EDGE ( 'NONE', *, *, #1597, .F. ) ;
#11140=VECTOR ( 'NONE', #3018, 1000.000000000000114 ) ;
#11148=CARTESIAN_POINT ( 'NONE',  ( -4.030227849471724966, 38.50929569396286212, -29.00044198939601969 ) ) ;
#11153=EDGE_CURVE ( 'NONE', #19223, #8379, #16997, .T. ) ;
#11158=DIRECTION ( 'NONE',  ( -1.000000000000000000, 0.000000000000000000, 0.000000000000000000 ) ) ;
#11163=DIRECTION ( 'NONE',  ( 0.000000000000000000, -1.000000000000000000, 0.000000000000000000 ) ) ;
#11165=CARTESIAN_POINT ( 'NONE',  ( 3.000000000291852764, 42.99999999900385461, -18.50000000000000355 ) ) ;
#11172=VECTOR ( 'NONE', #15600, 1000.000000000000114 ) ;
#11186=CARTESIAN_POINT ( 'NONE',  ( 36.00000000029184832, 2.999999999003851503, -39.00000000000000000 ) ) ;
#11188=TOROIDAL_SURFACE ( 'NONE', #301, 1.000000000000000000, 0.5000000000000000000 ) ;
#11196=CARTESIAN_POINT ( 'NONE',  ( 6.000000000291855429, -9.961476088449217059E-10, -3.449999999999997957 ) ) ;
#11207=UNCERTAINTY_MEASURE_WITH_UNIT (LENGTH_MEASURE( 1.000000000000000082E-05 ), #17292, 'distance_accuracy_value', 'NONE');
#11224=CARTESIAN_POINT ( 'NONE',  ( 2.918498775983380256E-10, 2.999999999003851503, -45.00000000000000000 ) ) ;
#11232=ORIENTED_EDGE ( 'NONE', *, *, #4707, .T. ) ;
#11242=EDGE_CURVE ( 'NONE', #15365, #15655, #4875, .T. ) ;
#11243=CARTESIAN_POINT ( 'NONE',  ( 36.00000000029184832, 2.999999999003851503, -18.50000000000000355 ) ) ;
#11259=DIRECTION ( 'NONE',  ( 1.000000000000000000, 0.000000000000000000, 0.000000000000000000 ) ) ;
#11276=DIRECTION ( 'NONE',  ( 1.000000000000000000, 0.000000000000000000, 0.000000000000000000 ) ) ;
#11290=CARTESIAN_POINT ( 'NONE',  ( 0.4500000002918510544, 42.99999999900385461, -26.00000000000000000 ) ) ;
#11307=ADVANCED_FACE ( 'NONE', ( #8885 ), #13828, .F. ) ;
#11328=CIRCLE ( 'NONE', #2687, 6.999999999999999112 ) ;
#11338=ORIENTED_EDGE ( 'NONE', *, *, #2930, .T. ) ;
#11339=ORIENTED_EDGE ( 'NONE', *, *, #20909, .F. ) ;
#11344=CARTESIAN_POINT ( 'NONE',  ( -3.999999999708153453, 38.99999999900385461, -15.99999999999999289 ) ) ;
#11352=DIRECTION ( 'NONE',  ( -0.000000000000000000, -1.000000000000000000, -0.000000000000000000 ) ) ;
#11408=CARTESIAN_POINT ( 'NONE',  ( -4.499999999708154341, 36.49999999900384751, -26.00000000000000000 ) ) ;
#11412=DIRECTION ( 'NONE',  ( -0.000000000000000000, 1.000000000000000000, 0.000000000000000000 ) ) ;
#11415=AXIS2_PLACEMENT_3D ( 'NONE', #19112, #17224, #6190 ) ;
#11417=CARTESIAN_POINT ( 'NONE',  ( -6.649675532656707411, 36.01889503913411517, -17.57202100271285872 ) ) ;
#11427=DIRECTION ( 'NONE',  ( 0.000000000000000000, 0.000000000000000000, 1.000000000000000000 ) ) ;
#11428=ORIENTED_EDGE ( 'NONE', *, *, #10672, .T. ) ;
#11451=ADVANCED_FACE ( 'NONE', ( #21943 ), #4043, .F. ) ;
#11454=CARTESIAN_POINT ( 'NONE',  ( -4.920724633012840243, 13.68667664578917709, -28.86177711096811649 ) ) ;
#11457=VERTEX_POINT ( 'NONE', #11798 ) ;
#11475=DIRECTION ( 'NONE',  ( -0.000000000000000000, -1.000000000000000000, -0.000000000000000000 ) ) ;
#11506=CARTESIAN_POINT ( 'NONE',  ( -3.999999999708153453, 35.49999999900384751, -25.50000000000000000 ) ) ;
#11507=ADVANCED_FACE ( 'NONE', ( #16851 ), #20641, .F. ) ;
#11525=DIRECTION ( 'NONE',  ( -0.000000000000000000, 1.000000000000000000, -0.000000000000000000 ) ) ;
#11527=CARTESIAN_POINT ( 'NONE',  ( -4.030227849471724078, 38.50929569396286212, -15.99955801060398031 ) ) ;
#11533=EDGE_CURVE ( 'NONE', #13010, #688, #8757, .T. ) ;
#11539=DIRECTION ( 'NONE',  ( 0.000000000000000000, 0.000000000000000000, 1.000000000000000000 ) ) ;
#11562=CARTESIAN_POINT ( 'NONE',  ( 3.000000000291852764, 42.99999999900385461, -19.00000000000000355 ) ) ;
#11570=CARTESIAN_POINT ( 'NONE',  ( -6.899936419963479395, 13.99939863585067990, -26.79405629275723655 ) ) ;
#11580=ORIENTED_EDGE ( 'NONE', *, *, #19442, .T. ) ;
#11597=CARTESIAN_POINT ( 'NONE',  ( 30.00000000029184832, -9.961476088449217059E-10, -5.999999999999998224 ) ) ;
#11606=ORIENTED_EDGE ( 'NONE', *, *, #17181, .T. ) ;
#11611=ORIENTED_EDGE ( 'NONE', *, *, #2195, .T. ) ;
#11616=CARTESIAN_POINT ( 'NONE',  ( -4.550510256924972907, 36.49999999900384751, -19.00000000000000355 ) ) ;
#11649=DIRECTION ( 'NONE',  ( 0.000000000000000000, -1.000000000000000000, 0.000000000000000000 ) ) ;
#11671=DIRECTION ( 'NONE',  ( 0.000000000000000000, 0.000000000000000000, 1.000000000000000000 ) ) ;
#11673=DIRECTION ( 'NONE',  ( 0.000000000000000000, 0.000000000000000000, -1.000000000000000000 ) ) ;
#11697=CIRCLE ( 'NONE', #21856, 7.000000000000006217 ) ;
#11705=DIRECTION ( 'NONE',  ( -0.000000000000000000, -0.000000000000000000, -1.000000000000000000 ) ) ;
#11714=DIRECTION ( 'NONE',  ( -1.000000000000000000, 0.000000000000000000, 0.000000000000000000 ) ) ;
#11718=ORIENTED_EDGE ( 'NONE', *, *, #12246, .T. ) ;
#11725=CARTESIAN_POINT ( 'NONE',  ( -4.499999999708154341, 35.49999999900384751, -19.50000000000000355 ) ) ;
#11739=AXIS2_PLACEMENT_3D ( 'NONE', #18736, #22153, #2388 ) ;
#11740=CARTESIAN_POINT ( 'NONE',  ( 35.50000000029185543, 16.99999999900385461, -26.00000000000000000 ) ) ;
#11746=CARTESIAN_POINT ( 'NONE',  ( 2.918498775983380256E-10, 2.999999999003851503, -26.00000000000000000 ) ) ;
#11750=EDGE_LOOP ( 'NONE', ( #19467, #12087, #22707, #5489 ) ) ;
#11759=DIRECTION ( 'NONE',  ( 1.000000000000000000, 0.000000000000000000, 0.000000000000000000 ) ) ;
#11783=EDGE_LOOP ( 'NONE', ( #18268, #13303, #250, #17904 ) ) ;
#11798=CARTESIAN_POINT ( 'NONE',  ( -6.959810536856680940, 36.00015702695179698, -26.48940942388196618 ) ) ;
#11824=CARTESIAN_POINT ( 'NONE',  ( 36.00000000029184832, 5.999999999003851059, -28.99999999999999645 ) ) ;
#11829=DIRECTION ( 'NONE',  ( 0.000000000000000000, 0.000000000000000000, -1.000000000000000000 ) ) ;
#11838=ADVANCED_FACE ( 'NONE', ( #7330 ), #16360, .F. ) ;
#11842=CARTESIAN_POINT ( 'NONE',  ( -3.999999999708153453, 13.99999999900385106, -22.50000000000000000 ) ) ;
#11848=VERTEX_POINT ( 'NONE', #8578 ) ;
#11855=DIRECTION ( 'NONE',  ( -0.000000000000000000, -0.000000000000000000, 1.000000000000000000 ) ) ;
#11858=CARTESIAN_POINT ( 'NONE',  ( -6.130979318160965086, 35.99999999900384040, -18.86947933461498295 ) ) ;
#11863=AXIS2_PLACEMENT_3D ( 'NONE', #21093, #4959, #14025 ) ;
#11883=DIRECTION ( 'NONE',  ( 0.000000000000000000, 0.000000000000000000, -1.000000000000000000 ) ) ;
#11887=CARTESIAN_POINT ( 'NONE',  ( 30.00000000029184832, 2.999999999003851503, -39.00000000000000000 ) ) ;
#11894=ORIENTED_EDGE ( 'NONE', *, *, #17331, .F. ) ;
#11944=ORIENTED_EDGE ( 'NONE', *, *, #12894, .F. ) ;
#11949=PLANE ( 'NONE',  #20572 ) ;
#11951=ADVANCED_FACE ( 'NONE', ( #17629 ), #5972, .F. ) ;
#11966=CARTESIAN_POINT ( 'NONE',  ( -6.958039891257955745, 36.00029345514013102, -26.50000000000000000 ) ) ;
#11988=FACE_OUTER_BOUND ( 'NONE', #11783, .T. ) ;
#11993=FACE_OUTER_BOUND ( 'NONE', #22672, .T. ) ;
#12015=CYLINDRICAL_SURFACE ( 'NONE', #11863, 2.550000000000003819 ) ;
#12033=ORIENTED_EDGE ( 'NONE', *, *, #14696, .F. ) ;
#12035=ORIENTED_EDGE ( 'NONE', *, *, #15004, .T. ) ;
#12041=ORIENTED_EDGE ( 'NONE', *, *, #20662, .T. ) ;
#12042=CARTESIAN_POINT ( 'NONE',  ( 30.00000000029184832, 2.999999999003851503, -41.54999999999999716 ) ) ;
#12052=EDGE_LOOP ( 'NONE', ( #4779, #2611, #13734, #20379 ) ) ;
#12053=DIRECTION ( 'NONE',  ( -0.000000000000000000, 1.000000000000000000, -0.000000000000000000 ) ) ;
#12054=FACE_OUTER_BOUND ( 'NONE', #17070, .T. ) ;
#12057=ORIENTED_EDGE ( 'NONE', *, *, #7643, .T. ) ;
#12059=AXIS2_PLACEMENT_3D ( 'NONE', #11033, #13036, #7624 ) ;
#12061=ADVANCED_FACE ( 'NONE', ( #15250 ), #9530, .F. ) ;
#12065=DIRECTION ( 'NONE',  ( 0.000000000000000000, 0.000000000000000000, -1.000000000000000000 ) ) ;
#12068=FACE_OUTER_BOUND ( 'NONE', #15425, .T. ) ;
#12078=CARTESIAN_POINT ( 'NONE',  ( -4.550510256924974684, 36.49999999900384751, -26.00000000000000000 ) ) ;
#12085=CARTESIAN_POINT ( 'NONE',  ( -4.775149780310945502, 35.99999999900384751, -25.50000003196489118 ) ) ;
#12087=ORIENTED_EDGE ( 'NONE', *, *, #4642, .T. ) ;
#12092=ORIENTED_EDGE ( 'NONE', *, *, #10925, .F. ) ;
#12096=CARTESIAN_POINT ( 'NONE',  ( -5.350349885510701675, 36.24720445779460931, -26.09137067849287206 ) ) ;
#12098=ORIENTED_EDGE ( 'NONE', *, *, #21021, .T. ) ;
#12104=ADVANCED_FACE ( 'NONE', ( #6915 ), #9024, .T. ) ;
#12105=DIRECTION ( 'NONE',  ( 0.7071067811865474617, -0.7071067811865474617, 0.000000000000000000 ) ) ;
#12113=FILL_AREA_STYLE ('',( #8840 ) ) ;
#12125=VERTEX_POINT ( 'NONE', #4895 ) ;
#12126=ORIENTED_EDGE ( 'NONE', *, *, #12128, .T. ) ;
#12128=EDGE_CURVE ( 'NONE', #8379, #4761, #12542, .T. ) ;
#12131=CARTESIAN_POINT ( 'NONE',  ( 6.000000000291855429, -0.5000000009961480529, -5.999999999999998224 ) ) ;
#12141=FACE_OUTER_BOUND ( 'NONE', #8262, .T. ) ;
#12146=CARTESIAN_POINT ( 'NONE',  ( 30.00000000029184832, -9.961476088449217059E-10, -5.999999999999998224 ) ) ;
#12152=VERTEX_POINT ( 'NONE', #12305 ) ;
#12166=VECTOR ( 'NONE', #4008, 1000.000000000000000 ) ;
#12168=VECTOR ( 'NONE', #7331, 1000.000000000000000 ) ;
#12185=EDGE_LOOP ( 'NONE', ( #13610, #20863, #2852, #4314 ) ) ;
#12191=DIRECTION ( 'NONE',  ( 0.000000000000000000, 1.000000000000000000, 0.000000000000000000 ) ) ;
#12192=FACE_BOUND ( 'NONE', #22418, .T. ) ;
#12206=CARTESIAN_POINT ( 'NONE',  ( -5.631870895226652962, 35.99999999900384751, -25.73470486101134469 ) ) ;
#12207=VERTEX_POINT ( 'NONE', #13850 ) ;
#12234=EDGE_LOOP ( 'NONE', ( #3462, #10621, #23242, #13181 ) ) ;
#12236=ORIENTED_EDGE ( 'NONE', *, *, #21821, .F. ) ;
#12246=EDGE_CURVE ( 'NONE', #3554, #283, #12776, .T. ) ;
#12247=DIRECTION ( 'NONE',  ( 0.000000000000000000, 0.000000000000000000, -1.000000000000000000 ) ) ;
#12266=ORIENTED_EDGE ( 'NONE', *, *, #4461, .T. ) ;
#12273=AXIS2_PLACEMENT_3D ( 'NONE', #15407, #21405, #13540 ) ;
#12277=DIRECTION ( 'NONE',  ( -1.000000000000000000, -0.000000000000000000, -0.000000000000000000 ) ) ;
#12287=CIRCLE ( 'NONE', #12681, 2.550000000000003819 ) ;
#12289=ADVANCED_FACE ( 'NONE', ( #10887 ), #16406, .T. ) ;
#12290=CARTESIAN_POINT ( 'NONE',  ( -3.499999999708153453, 2.999999999003851503, -19.00000000000000355 ) ) ;
#12294=CARTESIAN_POINT ( 'NONE',  ( -3.999999999708139686, 13.32455531934060744, -29.00000000000000355 ) ) ;
#12296=VERTEX_POINT ( 'NONE', #7377 ) ;
#12305=CARTESIAN_POINT ( 'NONE',  ( 35.50000000029184832, -9.961476088449217059E-10, -26.00000000000000000 ) ) ;
#12311=DIRECTION ( 'NONE',  ( 0.000000000000000000, 1.000000000000000000, 0.000000000000000000 ) ) ;
#12314=DIRECTION ( 'NONE',  ( 0.000000000000000000, 0.000000000000000000, 1.000000000000000000 ) ) ;
#12315=DIRECTION ( 'NONE',  ( 0.000000000000000000, 0.000000000000000000, 1.000000000000000000 ) ) ;
#12325=EDGE_LOOP ( 'NONE', ( #16976, #6419 ) ) ;
#12327=CARTESIAN_POINT ( 'NONE',  ( -4.550510256924972907, 36.49999999900384751, -26.00000000000000000 ) ) ;
#12336=CARTESIAN_POINT ( 'NONE',  ( -6.999999999708156118, 6.999999999003851947, -19.00000000000000355 ) ) ;
#12347=CARTESIAN_POINT ( 'NONE',  ( 2.918498775983380256E-10, -9.961476088449217059E-10, 0.000000000000000000 ) ) ;
#12358=ORIENTED_EDGE ( 'NONE', *, *, #3629, .F. ) ;
#12376=EDGE_CURVE ( 'NONE', #8151, #15365, #13015, .T. ) ;
#12387=VERTEX_POINT ( 'NONE', #4066 ) ;
#12389=ADVANCED_FACE ( 'NONE', ( #206 ), #1296, .T. ) ;
#12405=CARTESIAN_POINT ( 'NONE',  ( 2.918498775983380256E-10, 6.999999999003851947, -26.00000000000000000 ) ) ;
#12432=DIRECTION ( 'NONE',  ( -0.000000000000000000, 1.000000000000000000, -0.000000000000000000 ) ) ;
#12440=CARTESIAN_POINT ( 'NONE',  ( 7.596194078004423034, 47.59619407671642222, -26.00000000000000000 ) ) ;
#12443=VERTEX_POINT ( 'NONE', #2767 ) ;
#12446=CARTESIAN_POINT ( 'NONE',  ( -6.525563119727650907, 36.00216957434302856, -26.37497832018746280 ) ) ;
#12447=EDGE_LOOP ( 'NONE', ( #1127, #7399, #4421, #4721, #16084, #16112, #11611 ) ) ;
#12458=DIRECTION ( 'NONE',  ( 1.000000000000000000, 0.000000000000000000, 0.000000000000000000 ) ) ;
#12466=FACE_OUTER_BOUND ( 'NONE', #983, .T. ) ;
#12473=EDGE_LOOP ( 'NONE', ( #1720, #9787, #21369, #16260, #3430, #13094, #23020 ) ) ;
#12476=CARTESIAN_POINT ( 'NONE',  ( -3.999999999708139686, 49.99999999900385461, -18.99999999999998934 ) ) ;
#12479=CIRCLE ( 'NONE', #13229, 2.550000000000002043 ) ;
#12482=LINE ( 'NONE', #7210, #5754 ) ;
#12489=CARTESIAN_POINT ( 'NONE',  ( 26.45000000029184051, 16.99999999900385461, -19.49999999999998934 ) ) ;
#12490=AXIS2_PLACEMENT_3D ( 'NONE', #16043, #21372, #1820 ) ;
#12493=DIRECTION ( 'NONE',  ( 0.000000000000000000, 0.000000000000000000, -1.000000000000000000 ) ) ;
#12498=EDGE_CURVE ( 'NONE', #3520, #84, #14066, .T. ) ;
#12507=B_SPLINE_CURVE_WITH_KNOTS ( 'NONE', 3,
 ( #1142, #8432, #19474, #8770 ),
 .UNSPECIFIED., .F., .F.,
 ( 4, 4 ),
 ( 0.000000000000000000, 1.361771040845327923E-05 ),
 .UNSPECIFIED. ) ;
#12517=DIRECTION ( 'NONE',  ( -0.000000000000000000, -0.000000000000000000, 1.000000000000000000 ) ) ;
#12525=CARTESIAN_POINT ( 'NONE',  ( -6.230270079314315979, 13.95903802731504584, -16.98373150477994287 ) ) ;
#12531=TOROIDAL_SURFACE ( 'NONE', #9151, 6.500000000000005329, 0.5000000000000000000 ) ;
#12542=LINE ( 'NONE', #21394, #18545 ) ;
#12544=AXIS2_PLACEMENT_3D ( 'NONE', #15086, #22051, #2284 ) ;
#12550=FACE_BOUND ( 'NONE', #16397, .T. ) ;
#12553=EDGE_CURVE ( 'NONE', #12207, #14170, #21218, .T. ) ;
#12562=CIRCLE ( 'NONE', #1670, 0.5000000000000004441 ) ;
#12566=ADVANCED_FACE ( 'NONE', ( #6643 ), #15799, .F. ) ;
#12567=AXIS2_PLACEMENT_3D ( 'NONE', #15076, #10033, #8275 ) ;
#12571=CARTESIAN_POINT ( 'NONE',  ( -4.720100440588442581, 36.44386358680064575, -26.00000000000000000 ) ) ;
#12574=CARTESIAN_POINT ( 'NONE',  ( 30.00000000029184832, 2.999999999003851503, -45.00000000000000000 ) ) ;
#12582=CARTESIAN_POINT ( 'NONE',  ( -6.999999999708142795, 13.99999999900385106, -26.00000000000000000 ) ) ;
#12589=ORIENTED_EDGE ( 'NONE', *, *, #14098, .T. ) ;
#12596=ADVANCED_FACE ( 'NONE', ( #14292 ), #17689, .T. ) ;
#12603=AXIS2_PLACEMENT_3D ( 'NONE', #17729, #5150, #12314 ) ;
#12611=LINE ( 'NONE', #16134, #6310 ) ;
#12614=DIRECTION ( 'NONE',  ( -1.000000000000000000, 0.000000000000000000, -0.000000000000000000 ) ) ;
#12628=ORIENTED_EDGE ( 'NONE', *, *, #19414, .T. ) ;
#12641=CARTESIAN_POINT ( 'NONE',  ( -6.999999999708142795, 38.99999999900385461, -22.50000000000000000 ) ) ;
#12646=LINE ( 'NONE', #17598, #19498 ) ;
#12647=VERTEX_POINT ( 'NONE', #1577 ) ;
#12648=ORIENTED_EDGE ( 'NONE', *, *, #9405, .F. ) ;
#12654=ORIENTED_EDGE ( 'NONE', *, *, #1787, .T. ) ;
#12667=VECTOR ( 'NONE', #23085, 1000.000000000000000 ) ;
#12681=AXIS2_PLACEMENT_3D ( 'NONE', #14811, #2338, #16787 ) ;
#12685=EDGE_CURVE ( 'NONE', #1665, #8753, #8760, .T. ) ;
#12710=ORIENTED_EDGE ( 'NONE', *, *, #3258, .F. ) ;
#12735=CARTESIAN_POINT ( 'NONE',  ( -6.590924991943732714, 35.99999999900384751, -18.75864816872293162 ) ) ;
#12740=VERTEX_POINT ( 'NONE', #7576 ) ;
#12745=AXIS2_PLACEMENT_3D ( 'NONE', #18314, #2192, #21966 ) ;
#12759=FACE_OUTER_BOUND ( 'NONE', #7368, .T. ) ;
#12776=LINE ( 'NONE', #11344, #19677 ) ;
#12810=DIRECTION ( 'NONE',  ( 0.000000000000000000, 0.000000000000000000, 1.000000000000000000 ) ) ;
#12824=ORIENTED_EDGE ( 'NONE', *, *, #22576, .T. ) ;
#12826=ADVANCED_FACE ( 'NONE', ( #12866 ), #20052, .T. ) ;
#12832=LINE ( 'NONE', #2120, #3947 ) ;
#12837=MANIFOLD_SOLID_BREP ( 'Fillet12', #4289 ) ;
#12838=CARTESIAN_POINT ( 'NONE',  ( -6.846097631013046581, 36.00232955766364285, -18.02039154777020613 ) ) ;
#12859=ADVANCED_FACE ( 'NONE', ( #987 ), #13337, .F. ) ;
#12863=FACE_OUTER_BOUND ( 'NONE', #4142, .T. ) ;
#12866=FACE_OUTER_BOUND ( 'NONE', #13211, .T. ) ;
#12867=EDGE_CURVE ( 'NONE', #20043, #14311, #13452, .T. ) ;
#12875=CARTESIAN_POINT ( 'NONE',  ( -3.999999999708153453, 35.99999999900384751, -29.50000000000000000 ) ) ;
#12877=CARTESIAN_POINT ( 'NONE',  ( -3.499999999708153453, 13.99999999900385106, -25.50000000000000000 ) ) ;
#12884=TOROIDAL_SURFACE ( 'NONE', #3500, 6.500000000000005329, 0.5000000000000000000 ) ;
#12894=EDGE_CURVE ( 'NONE', #5703, #3643, #4846, .T. ) ;
#12907=CARTESIAN_POINT ( 'NONE',  ( -3.499999999708153453, 42.99999999900385461, -26.50000000000000000 ) ) ;
#12913=CARTESIAN_POINT ( 'NONE',  ( 29.00000000029184832, 16.99999999900385461, -15.99999999999999289 ) ) ;
#12918=ORIENTED_EDGE ( 'NONE', *, *, #5486, .T. ) ;
#12920=CARTESIAN_POINT ( 'NONE',  ( -5.784122180648308742, 36.25568647312941550, -28.41463637942309362 ) ) ;
#12931=CARTESIAN_POINT ( 'NONE',  ( 30.00000000029184832, 2.999999999003851503, -39.00000000000000000 ) ) ;
#12993=CIRCLE ( 'NONE', #5112, 2.999999999999999112 ) ;
#12998=CARTESIAN_POINT ( 'NONE',  ( 7.596194078004423034, 47.59619407671642222, -19.00000000000000355 ) ) ;
#13002=CIRCLE ( 'NONE', #10723, 0.5000000000000004441 ) ;
#13010=VERTEX_POINT ( 'NONE', #22857 ) ;
#13013=VECTOR ( 'NONE', #21167, 1000.000000000000000 ) ;
#13015=LINE ( 'NONE', #11243, #17834 ) ;
#13021=CARTESIAN_POINT ( 'NONE',  ( -6.958039891257955745, 36.00029345514013102, -18.49999999999999645 ) ) ;
#13022=ADVANCED_FACE ( 'NONE', ( #14142 ), #6734, .F. ) ;
#13029=EDGE_CURVE ( 'NONE', #1520, #19813, #21220, .T. ) ;
#13031=FACE_OUTER_BOUND ( 'NONE', #9909, .T. ) ;
#13035=CARTESIAN_POINT ( 'NONE',  ( -6.917363703046245149, 36.00086243655339757, -26.74064357473281817 ) ) ;
#13036=DIRECTION ( 'NONE',  ( -1.000000000000000000, 0.000000000000000000, 0.000000000000000000 ) ) ;
#13037=ORIENTED_EDGE ( 'NONE', *, *, #18243, .F. ) ;
#13041=AXIS2_PLACEMENT_3D ( 'NONE', #17180, #622, #4484 ) ;
#13048=ADVANCED_FACE ( 'NONE', ( #5319 ), #12531, .T. ) ;
#13061=EDGE_LOOP ( 'NONE', ( #3175, #15215 ) ) ;
#13064=VECTOR ( 'NONE', #1451, 1000.000000000000000 ) ;
#13069=DIRECTION ( 'NONE',  ( 0.000000000000000000, -1.000000000000000000, 0.000000000000000000 ) ) ;
#13074=CIRCLE ( 'NONE', #1066, 2.550000000000003819 ) ;
#13075=DIRECTION ( 'NONE',  ( 0.000000000000000000, -1.000000000000000000, 0.000000000000000000 ) ) ;
#13082=CIRCLE ( 'NONE', #17979, 6.500000000000000888 ) ;
#13094=ORIENTED_EDGE ( 'NONE', *, *, #10356, .F. ) ;
#13097=VERTEX_POINT ( 'NONE', #11408 ) ;
#13102=AXIS2_PLACEMENT_3D ( 'NONE', #5599, #9462, #412 ) ;
#13127=ADVANCED_FACE ( 'NONE', ( #4467 ), #4116, .T. ) ;
#13128=ORIENTED_EDGE ( 'NONE', *, *, #15004, .F. ) ;
#13133=DIRECTION ( 'NONE',  ( 0.000000000000000000, 0.000000000000000000, -1.000000000000000000 ) ) ;
#13149=EDGE_CURVE ( 'NONE', #7942, #690, #4578, .T. ) ;
#13153=ORIENTED_EDGE ( 'NONE', *, *, #8818, .T. ) ;
#13156=EDGE_CURVE ( 'NONE', #8964, #3689, #14831, .T. ) ;
#13157=CARTESIAN_POINT ( 'NONE',  ( -6.846097631013046581, 36.00232955766364285, -26.97960845222978676 ) ) ;
#13160=VECTOR ( 'NONE', #989, 1000.000000000000000 ) ;
#13166=ADVANCED_FACE ( 'NONE', ( #20253 ), #18474, .T. ) ;
#13181=ORIENTED_EDGE ( 'NONE', *, *, #14696, .T. ) ;
#13192=DIRECTION ( 'NONE',  ( -0.000000000000000000, 1.000000000000000000, -0.000000000000000000 ) ) ;
#13202=ORIENTED_EDGE ( 'NONE', *, *, #4114, .F. ) ;
#13206=VERTEX_POINT ( 'NONE', #6823 ) ;
#13211=EDGE_LOOP ( 'NONE', ( #1722, #2898, #3290, #5928 ) ) ;
#13212=SURFACE_STYLE_FILL_AREA ( #18739 ) ;
#13219=AXIS2_PLACEMENT_3D ( 'NONE', #7724, #4073, #7954 ) ;
#13223=EDGE_CURVE ( 'NONE', #11457, #21236, #2244, .T. ) ;
#13229=AXIS2_PLACEMENT_3D ( 'NONE', #22984, #15667, #2865 ) ;
#13231=ORIENTED_EDGE ( 'NONE', *, *, #5455, .T. ) ;
#13259=ADVANCED_FACE ( 'NONE', ( #11988 ), #13654, .F. ) ;
#13270=EDGE_LOOP ( 'NONE', ( #15675, #18731, #8644, #14284 ) ) ;
#13271=AXIS2_PLACEMENT_3D ( 'NONE', #10816, #3538, #14000 ) ;
#13295=AXIS2_PLACEMENT_3D ( 'NONE', #18233, #7411, #11276 ) ;
#13299=CIRCLE ( 'NONE', #4259, 7.000000000000000000 ) ;
#13301=ORIENTED_EDGE ( 'NONE', *, *, #16707, .F. ) ;
#13303=ORIENTED_EDGE ( 'NONE', *, *, #19341, .T. ) ;
#13313=CARTESIAN_POINT ( 'NONE',  ( -4.938244945965066357, 36.80742465210828840, -16.14556293119101937 ) ) ;
#13317=EDGE_CURVE ( 'NONE', #2802, #4871, #10469, .T. ) ;
#13327=ORIENTED_EDGE ( 'NONE', *, *, #15193, .F. ) ;
#13337=CYLINDRICAL_SURFACE ( 'NONE', #12567, 0.5000000000000004441 ) ;
#13340=DIRECTION ( 'NONE',  ( 0.000000000000000000, 0.000000000000000000, -1.000000000000000000 ) ) ;
#13341=DIRECTION ( 'NONE',  ( 0.000000000000000000, 0.000000000000000000, 1.000000000000000000 ) ) ;
#13349=CARTESIAN_POINT ( 'NONE',  ( -4.733938537004359404, 13.62597557122357372, -28.91485355091821674 ) ) ;
#13362=ORIENTED_EDGE ( 'NONE', *, *, #6959, .F. ) ;
#13363=DIRECTION ( 'NONE',  ( 0.000000000000000000, 0.000000000000000000, -1.000000000000000000 ) ) ;
#13375=CIRCLE ( 'NONE', #2098, 0.5000000000000004441 ) ;
#13376=CYLINDRICAL_SURFACE ( 'NONE', #1090, 2.999999999999999112 ) ;
#13377=DIRECTION ( 'NONE',  ( 1.000000000000000000, 0.000000000000000000, 0.000000000000000000 ) ) ;
#13379=VECTOR ( 'NONE', #4911, 1000.000000000000000 ) ;
#13396=VECTOR ( 'NONE', #6776, 1000.000000000000000 ) ;
#13411=VERTEX_POINT ( 'NONE', #18228 ) ;
#13424=EDGE_CURVE ( 'NONE', #18888, #7942, #6741, .T. ) ;
#13425=LINE ( 'NONE', #9774, #1257 ) ;
#13448=CYLINDRICAL_SURFACE ( 'NONE', #9511, 2.550000000000003819 ) ;
#13452=LINE ( 'NONE', #20633, #19716 ) ;
#13460=CARTESIAN_POINT ( 'NONE',  ( 2.918498775983380256E-10, -9.961476088449217059E-10, -26.00000000000000000 ) ) ;
#13487=PLANE ( 'NONE',  #9698 ) ;
#13490=DIRECTION ( 'NONE',  ( 0.000000000000000000, 0.000000000000000000, -1.000000000000000000 ) ) ;
#13508=DIRECTION ( 'NONE',  ( -1.858632295689435609E-16, -1.000000000000000000, 0.000000000000000000 ) ) ;
#13523=LINE ( 'NONE', #15505, #13379 ) ;
#13537=CARTESIAN_POINT ( 'NONE',  ( 29.00000000029184832, 16.99999999900385461, -19.00000000000000355 ) ) ;
#13540=DIRECTION ( 'NONE',  ( 1.000000000000000000, 0.000000000000000000, 0.000000000000000000 ) ) ;
#13541=ADVANCED_FACE ( 'NONE', ( #9956 ), #15350, .F. ) ;
#13544=VECTOR ( 'NONE', #13340, 1000.000000000000000 ) ;
#13571=CARTESIAN_POINT ( 'NONE',  ( 36.00000000029184832, 2.999999999003851503, -45.00000000000000000 ) ) ;
#13578=CIRCLE ( 'NONE', #22589, 2.550000000000003819 ) ;
#13583=ORIENTED_EDGE ( 'NONE', *, *, #6779, .T. ) ;
#13598=ORIENTED_EDGE ( 'NONE', *, *, #325, .T. ) ;
#13610=ORIENTED_EDGE ( 'NONE', *, *, #13424, .T. ) ;
#13611=DIRECTION ( 'NONE',  ( 0.000000000000000000, 0.000000000000000000, -1.000000000000000000 ) ) ;
#13612=CARTESIAN_POINT ( 'NONE',  ( -6.999999999708142795, 38.99999999900385461, -18.50000000000000355 ) ) ;
#13613=CIRCLE ( 'NONE', #10219, 7.000000000000000000 ) ;
#13625=FACE_OUTER_BOUND ( 'NONE', #5982, .T. ) ;
#13628=CARTESIAN_POINT ( 'NONE',  ( -5.423466998247613802, 35.99999999900384751, -19.34679001651818098 ) ) ;
#13641=VERTEX_POINT ( 'NONE', #12042 ) ;
#13645=EDGE_LOOP ( 'NONE', ( #4949, #10634, #19343, #20276 ) ) ;
#13654=CYLINDRICAL_SURFACE ( 'NONE', #7, 6.999999999999999112 ) ;
#13663=VECTOR ( 'NONE', #14116, 1000.000000000000000 ) ;
#13680=CARTESIAN_POINT ( 'NONE',  ( 7.949747468597695210, 47.94974746730969173, -18.50000000000000355 ) ) ;
#13686=CARTESIAN_POINT ( 'NONE',  ( 33.94974746859769255, 21.94974746730969528, -19.49999999999998934 ) ) ;
#13689=ADVANCED_FACE ( 'NONE', ( #10290 ), #5356, .F. ) ;
#13700=DIRECTION ( 'NONE',  ( 0.000000000000000000, 0.000000000000000000, -1.000000000000000000 ) ) ;
#13708=ORIENTED_EDGE ( 'NONE', *, *, #6485, .T. ) ;
#13710=ORIENTED_EDGE ( 'NONE', *, *, #15820, .T. ) ;
#13715=DIRECTION ( 'NONE',  ( 0.000000000000000000, 0.000000000000000000, 1.000000000000000000 ) ) ;
#13720=CARTESIAN_POINT ( 'NONE',  ( -6.959810536856695151, 36.00015702695179698, -18.51059057611807646 ) ) ;
#13734=ORIENTED_EDGE ( 'NONE', *, *, #22202, .F. ) ;
#13751=DIRECTION ( 'NONE',  ( 0.000000000000000000, 1.000000000000000000, 0.000000000000000000 ) ) ;
#13753=CIRCLE ( 'NONE', #3606, 0.5000000000000004441 ) ;
#13759=EDGE_LOOP ( 'NONE', ( #2035, #9820, #13037, #2085 ) ) ;
#13761=ORIENTED_EDGE ( 'NONE', *, *, #22202, .T. ) ;
#13772=DIRECTION ( 'NONE',  ( -0.000000000000000000, -0.000000000000000000, 1.000000000000000000 ) ) ;
#13777=CARTESIAN_POINT ( 'NONE',  ( -6.999999999708142795, 35.99999999900384751, -26.00000000000000000 ) ) ;
#13786=ORIENTED_EDGE ( 'NONE', *, *, #13983, .F. ) ;
#13811=VECTOR ( 'NONE', #8226, 1000.000000000000000 ) ;
#13812=ORIENTED_EDGE ( 'NONE', *, *, #1597, .T. ) ;
#13828=PLANE ( 'NONE',  #12490 ) ;
#13829=CARTESIAN_POINT ( 'NONE',  ( 29.00000000029184832, 16.99999999900385461, -25.50000000000000355 ) ) ;
#13850=CARTESIAN_POINT ( 'NONE',  ( 5.550000000291854363, 42.99999999900385461, -15.99999999999999289 ) ) ;
#13853=DIRECTION ( 'NONE',  ( 1.000000000000000000, 0.000000000000000000, 0.000000000000000000 ) ) ;
#13854=LINE ( 'NONE', #19376, #19619 ) ;
#13855=VECTOR ( 'NONE', #13611, 1000.000000000000000 ) ;
#13856=EDGE_CURVE ( 'NONE', #8962, #8469, #20521, .T. ) ;
#13860=CARTESIAN_POINT ( 'NONE',  ( -3.999999999708153453, 42.99999999900385461, -26.50000000000000000 ) ) ;
#13867=CARTESIAN_POINT ( 'NONE',  ( 2.918498775983380256E-10, 2.999999999003851503, -19.00000000000000355 ) ) ;
#13872=EDGE_CURVE ( 'NONE', #7853, #7223, #15080, .T. ) ;
#13875=ORIENTED_EDGE ( 'NONE', *, *, #11242, .F. ) ;
#13917=DIRECTION ( 'NONE',  ( -1.000000000000000000, 0.000000000000000000, 0.000000000000000000 ) ) ;
#13929=DIRECTION ( 'NONE',  ( 0.000000000000000000, 0.000000000000000000, 1.000000000000000000 ) ) ;
#13942=CARTESIAN_POINT ( 'NONE',  ( -5.945013150601170970, 13.92153864138982300, -16.70732315498745635 ) ) ;
#13954=ORIENTED_EDGE ( 'NONE', *, *, #10933, .F. ) ;
#13962=CARTESIAN_POINT ( 'NONE',  ( 6.000000000291855429, 2.999999999003851503, -5.999999999999998224 ) ) ;
#13965=CARTESIAN_POINT ( 'NONE',  ( 36.00000000029184832, 5.999999999003851059, -32.00000000000000000 ) ) ;
#13967=DIRECTION ( 'NONE',  ( -0.000000000000000000, -0.000000000000000000, 1.000000000000000000 ) ) ;
#13974=CARTESIAN_POINT ( 'NONE',  ( 30.00000000029184832, -0.5000000009961480529, -36.45000000000000284 ) ) ;
#13980=EDGE_CURVE ( 'NONE', #12125, #18888, #18744, .T. ) ;
#13983=EDGE_CURVE ( 'NONE', #1430, #11848, #40, .T. ) ;
#14000=DIRECTION ( 'NONE',  ( 0.000000000000000000, 0.000000000000000000, -1.000000000000000000 ) ) ;
#14003=CIRCLE ( 'NONE', #18499, 2.550000000000003819 ) ;
#14012=VERTEX_POINT ( 'NONE', #3562 ) ;
#14022=AXIS2_PLACEMENT_3D ( 'NONE', #15619, #6233, #22351 ) ;
#14024=CIRCLE ( 'NONE', #8413, 6.999999999999999112 ) ;
#14025=DIRECTION ( 'NONE',  ( 1.000000000000000000, 0.000000000000000000, 0.000000000000000000 ) ) ;
#14063=CARTESIAN_POINT ( 'NONE',  ( -4.499999999708154341, 35.49999999900384751, -19.00000000000000355 ) ) ;
#14065=CARTESIAN_POINT ( 'NONE',  ( 29.00000000029184832, 16.99999999900385461, -15.99999999999999289 ) ) ;
#14066=CIRCLE ( 'NONE', #20082, 6.000000000000000000 ) ;
#14071=LINE ( 'NONE', #12290, #13396 ) ;
#14083=DIRECTION ( 'NONE',  ( -1.858632295689435609E-16, -1.000000000000000000, -2.999267978177796234E-32 ) ) ;
#14090=DIRECTION ( 'NONE',  ( 0.000000000000000000, 0.000000000000000000, -1.000000000000000000 ) ) ;
#14091=DIRECTION ( 'NONE',  ( -0.000000000000000000, 1.000000000000000000, -0.000000000000000000 ) ) ;
#14098=EDGE_CURVE ( 'NONE', #4567, #4761, #15891, .T. ) ;
#14104=CARTESIAN_POINT ( 'NONE',  ( -6.083292711281922394, 36.06725630338630140, -26.25729431478694664 ) ) ;
#14116=DIRECTION ( 'NONE',  ( 0.000000000000000000, -0.000000000000000000, -1.000000000000000000 ) ) ;
#14127=DIRECTION ( 'NONE',  ( 0.000000000000000000, 0.000000000000000000, -1.000000000000000000 ) ) ;
#14128=SURFACE_SIDE_STYLE ('',( #22961 ) ) ;
#14138=ORIENTED_EDGE ( 'NONE', *, *, #15256, .T. ) ;
#14142=FACE_OUTER_BOUND ( 'NONE', #11750, .T. ) ;
#14143=DIRECTION ( 'NONE',  ( 0.000000000000000000, 0.000000000000000000, 1.000000000000000000 ) ) ;
#14154=CIRCLE ( 'NONE', #2114, 7.000000000000006217 ) ;
#14170=VERTEX_POINT ( 'NONE', #1891 ) ;
#14180=CARTESIAN_POINT ( 'NONE',  ( -4.499999999708154341, 36.49999999900384751, -19.00000000000000355 ) ) ;
#14187=CARTESIAN_POINT ( 'NONE',  ( -4.182466315668081691, 13.41110669254460852, -15.99999999999999289 ) ) ;
#14192=DIRECTION ( 'NONE',  ( -1.000000000000000000, -0.000000000000000000, -1.613696256722611405E-16 ) ) ;
#14201=VERTEX_POINT ( 'NONE', #16123 ) ;
#14214=CARTESIAN_POINT ( 'NONE',  ( 6.000000000291855429, -9.961476088449217059E-10, -39.00000000000000000 ) ) ;
#14217=CYLINDRICAL_SURFACE ( 'NONE', #4412, 2.550000000000002043 ) ;
#14218=CIRCLE ( 'NONE', #1036, 3.500000000000000000 ) ;
#14244=CARTESIAN_POINT ( 'NONE',  ( -3.999999999708139686, 13.32455531934060744, -15.99999999999999289 ) ) ;
#14247=EDGE_CURVE ( 'NONE', #13411, #13010, #18372, .T. ) ;
#14256=VERTEX_POINT ( 'NONE', #9198 ) ;
#14257=EDGE_LOOP ( 'NONE', ( #17484, #10425, #12236, #10602, #14365, #21392, #4494 ) ) ;
#14272=CARTESIAN_POINT ( 'NONE',  ( 6.000000000291855429, 2.999999999003851503, -39.00000000000000000 ) ) ;
#14274=EDGE_CURVE ( 'NONE', #4090, #3970, #20016, .T. ) ;
#14284=ORIENTED_EDGE ( 'NONE', *, *, #12685, .F. ) ;
#14287=ORIENTED_EDGE ( 'NONE', *, *, #21934, .T. ) ;
#14292=FACE_OUTER_BOUND ( 'NONE', #695, .T. ) ;
#14293=ADVANCED_FACE ( 'NONE', ( #17050 ), #9892, .F. ) ;
#14303=EDGE_CURVE ( 'NONE', #3151, #18076, #8307, .T. ) ;
#14311=VERTEX_POINT ( 'NONE', #20848 ) ;
#14315=CIRCLE ( 'NONE', #5675, 0.5000000000000004441 ) ;
#14365=ORIENTED_EDGE ( 'NONE', *, *, #3421, .F. ) ;
#14369=VECTOR ( 'NONE', #845, 1000.000000000000000 ) ;
#14380=VECTOR ( 'NONE', #12517, 1000.000000000000000 ) ;
#14385=CARTESIAN_POINT ( 'NONE',  ( -4.550510256924974684, 35.99999999900384751, -19.50000000000000355 ) ) ;
#14387=ORIENTED_EDGE ( 'NONE', *, *, #21666, .F. ) ;
#14390=ORIENTED_EDGE ( 'NONE', *, *, #19414, .F. ) ;
#14393=ORIENTED_EDGE ( 'NONE', *, *, #9415, .T. ) ;
#14400=VECTOR ( 'NONE', #2651, 1000.000000000000000 ) ;
#14404=EDGE_LOOP ( 'NONE', ( #4917, #4751, #7904, #9981 ) ) ;
#14412=CARTESIAN_POINT ( 'NONE',  ( -4.499999999708154341, 36.49999999900384751, -25.50000000000000000 ) ) ;
#14436=AXIS2_PLACEMENT_3D ( 'NONE', #16045, #9234, #23254 ) ;
#14461=CARTESIAN_POINT ( 'NONE',  ( -3.999999999708153453, 38.99999999900385461, -29.00000000000000355 ) ) ;
#14471=CARTESIAN_POINT ( 'NONE',  ( 26.45000000029184051, 16.99999999900385461, -29.00000000000000355 ) ) ;
#14487=EDGE_LOOP ( 'NONE', ( #251, #4168, #4639, #10251 ) ) ;
#14500=ADVANCED_FACE ( 'NONE', ( #17763 ), #22956, .F. ) ;
#14517=DIRECTION ( 'NONE',  ( 1.000000000000000000, -0.000000000000000000, 0.000000000000000000 ) ) ;
#14521=DIRECTION ( 'NONE',  ( 1.000000000000000000, -1.858632295689435609E-16, 0.000000000000000000 ) ) ;
#14532=EDGE_CURVE ( 'NONE', #5983, #555, #14315, .T. ) ;
#14559=EDGE_LOOP ( 'NONE', ( #20511, #11034 ) ) ;
#14579=AXIS2_PLACEMENT_3D ( 'NONE', #8190, #11705, #18895 ) ;
#14613=CARTESIAN_POINT ( 'NONE',  ( 30.00000000029184832, -9.961476088449217059E-10, -36.45000000000000284 ) ) ;
#14619=ADVANCED_FACE ( 'NONE', ( #5765 ), #3981, .T. ) ;
#14621=VERTEX_POINT ( 'NONE', #14471 ) ;
#14634=ADVANCED_FACE ( 'NONE', ( #9288 ), #16335, .T. ) ;
#14653=VERTEX_POINT ( 'NONE', #12582 ) ;
#14655=VERTEX_POINT ( 'NONE', #18110 ) ;
#14682=DIRECTION ( 'NONE',  ( 1.613696256722611405E-16, -0.000000000000000000, -1.000000000000000000 ) ) ;
#14696=EDGE_CURVE ( 'NONE', #4926, #1834, #13578, .T. ) ;
#14699=VERTEX_POINT ( 'NONE', #356 ) ;
#14709=CARTESIAN_POINT ( 'NONE',  ( 35.50000000029184832, 16.99999999900385461, -18.50000000000000355 ) ) ;
#14722=DIRECTION ( 'NONE',  ( -0.000000000000000000, -0.000000000000000000, 1.000000000000000000 ) ) ;
#14735=ORIENTED_EDGE ( 'NONE', *, *, #15566, .F. ) ;
#14737=ORIENTED_EDGE ( 'NONE', *, *, #20882, .T. ) ;
#14749=CIRCLE ( 'NONE', #856, 2.550000000000000711 ) ;
#14752=DIRECTION ( 'NONE',  ( -1.000000000000000000, -0.000000000000000000, 0.000000000000000000 ) ) ;
#14779=CIRCLE ( 'NONE', #14436, 2.550000000000003819 ) ;
#14784=FACE_BOUND ( 'NONE', #22970, .T. ) ;
#14811=CARTESIAN_POINT ( 'NONE',  ( 29.00000000029184832, 16.99999999900385461, -26.00000000000000000 ) ) ;
#14819=FACE_BOUND ( 'NONE', #18764, .T. ) ;
#14820=AXIS2_PLACEMENT_3D ( 'NONE', #15208, #18863, #414 ) ;
#14831=LINE ( 'NONE', #5895, #9015 ) ;
#14892=CARTESIAN_POINT ( 'NONE',  ( 6.000000000291855429, -9.961476088449217059E-10, -41.55000000000000426 ) ) ;
#14916=DIRECTION ( 'NONE',  ( 1.858632295689435609E-16, 1.000000000000000000, 0.000000000000000000 ) ) ;
#14928=CARTESIAN_POINT ( 'NONE',  ( -6.999999999708142795, 35.99999999900384751, -22.50000000000000000 ) ) ;
#14931=VECTOR ( 'NONE', #2, 1000.000000000000000 ) ;
#14939=VECTOR ( 'NONE', #4047, 1000.000000000000000 ) ;
#14961=ORIENTED_EDGE ( 'NONE', *, *, #2313, .F. ) ;
#14963=VERTEX_POINT ( 'NONE', #13860 ) ;
#14966=EDGE_LOOP ( 'NONE', ( #1602, #2872, #1544, #22946 ) ) ;
#14976=CARTESIAN_POINT ( 'NONE',  ( -3.999999999708139686, 49.99999999900385461, -15.99999999999999289 ) ) ;
#14983=DIRECTION ( 'NONE',  ( 1.000000000000000000, 0.000000000000000000, 0.000000000000000000 ) ) ;
#14999=DIRECTION ( 'NONE',  ( 0.000000000000000000, -1.000000000000000000, 0.000000000000000000 ) ) ;
#15004=EDGE_CURVE ( 'NONE', #4543, #22761, #15806, .T. ) ;
#15014=FACE_BOUND ( 'NONE', #20997, .T. ) ;
#15044=ORIENTED_EDGE ( 'NONE', *, *, #12498, .T. ) ;
#15048=CARTESIAN_POINT ( 'NONE',  ( -3.499999999708153453, 35.99999999900384751, -18.50000000000000355 ) ) ;
#15051=CARTESIAN_POINT ( 'NONE',  ( -3.499999999708153453, 42.99999999900385461, -26.00000000000000000 ) ) ;
#15065=EDGE_CURVE ( 'NONE', #15111, #19572, #4931, .T. ) ;
#15076=CARTESIAN_POINT ( 'NONE',  ( 2.918498775983380256E-10, 36.49999999900384751, -25.50000000000000000 ) ) ;
#15080=LINE ( 'NONE', #13686, #13160 ) ;
#15086=CARTESIAN_POINT ( 'NONE',  ( 6.000000000291855429, 2.999999999003851503, -5.999999999999998224 ) ) ;
#15093=EDGE_CURVE ( 'NONE', #8753, #21236, #22971, .T. ) ;
#15096=EDGE_LOOP ( 'NONE', ( #6322, #2153, #2041, #28, #22949, #16376 ) ) ;
#15102=EDGE_CURVE ( 'NONE', #15655, #10116, #15116, .T. ) ;
#15110=DIRECTION ( 'NONE',  ( -0.000000000000000000, -0.000000000000000000, 1.000000000000000000 ) ) ;
#15111=VERTEX_POINT ( 'NONE', #22193 ) ;
#15116=LINE ( 'NONE', #6199, #4946 ) ;
#15131=FACE_BOUND ( 'NONE', #7691, .T. ) ;
#15135=ORIENTED_EDGE ( 'NONE', *, *, #6959, .T. ) ;
#15151=CARTESIAN_POINT ( 'NONE',  ( -4.904729001344796835, 35.99999999900385461, -19.07709762542843634 ) ) ;
#15157=CARTESIAN_POINT ( 'NONE',  ( -3.999999999708153453, 35.99999999900384751, -25.50000000000000000 ) ) ;
#15163=AXIS2_PLACEMENT_3D ( 'NONE', #11044, #2454, #5879 ) ;
#15176=VECTOR ( 'NONE', #1703, 1000.000000000000000 ) ;
#15193=EDGE_CURVE ( 'NONE', #20913, #8586, #19222, .T. ) ;
#15194=ORIENTED_EDGE ( 'NONE', *, *, #6779, .F. ) ;
#15199=DIRECTION ( 'NONE',  ( -1.000000000000000000, 0.000000000000000000, 0.000000000000000000 ) ) ;
#15200=EDGE_LOOP ( 'NONE', ( #1833, #21859, #22409, #11083 ) ) ;
#15208=CARTESIAN_POINT ( 'NONE',  ( -3.499999999708153453, 2.999999999003851503, -26.50000000000000000 ) ) ;
#15215=ORIENTED_EDGE ( 'NONE', *, *, #21476, .F. ) ;
#15223=CYLINDRICAL_SURFACE ( 'NONE', #19261, 2.549999999999996714 ) ;
#15250=FACE_OUTER_BOUND ( 'NONE', #21469, .T. ) ;
#15255=DIRECTION ( 'NONE',  ( -0.000000000000000000, -0.000000000000000000, 1.000000000000000000 ) ) ;
#15256=EDGE_CURVE ( 'NONE', #15655, #7223, #11697, .T. ) ;
#15260=DIRECTION ( 'NONE',  ( 0.000000000000000000, 0.000000000000000000, -1.000000000000000000 ) ) ;
#15261=VECTOR ( 'NONE', #9967, 1000.000000000000000 ) ;
#15276=AXIS2_PLACEMENT_3D ( 'NONE', #16713, #20375, #11539 ) ;
#15298=CARTESIAN_POINT ( 'NONE',  ( 6.000000000291855429, 2.999999999003851503, -45.00000000000000000 ) ) ;
#15308=ORIENTED_EDGE ( 'NONE', *, *, #4981, .F. ) ;
#15312=EDGE_LOOP ( 'NONE', ( #10058, #22024, #16488, #21926 ) ) ;
#15313=VECTOR ( 'NONE', #5507, 1000.000000000000114 ) ;
#15322=CARTESIAN_POINT ( 'NONE',  ( 0.4500000002918510544, 42.99999999900385461, -25.50000000000000355 ) ) ;
#15343=CIRCLE ( 'NONE', #5159, 7.000000000000006217 ) ;
#15345=ORIENTED_EDGE ( 'NONE', *, *, #16611, .T. ) ;
#15350=PLANE ( 'NONE',  #5272 ) ;
#15364=CARTESIAN_POINT ( 'NONE',  ( 36.00000000029184832, 2.999999999003851503, -5.999999999999998224 ) ) ;
#15365=VERTEX_POINT ( 'NONE', #21375 ) ;
#15366=ADVANCED_FACE ( 'NONE', ( #11072 ), #9552, .F. ) ;
#15368=VERTEX_POINT ( 'NONE', #12405 ) ;
#15376=DIRECTION ( 'NONE',  ( 1.000000000000000000, 0.000000000000000000, -0.000000000000000000 ) ) ;
#15392=AXIS2_PLACEMENT_3D ( 'NONE', #17464, #15691, #1364 ) ;
#15394=ORIENTED_EDGE ( 'NONE', *, *, #17181, .F. ) ;
#15399=CARTESIAN_POINT ( 'NONE',  ( 3.000000000291852764, 42.99999999900385461, -15.99999999999999289 ) ) ;
#15403=ORIENTED_EDGE ( 'NONE', *, *, #19611, .T. ) ;
#15405=DIRECTION ( 'NONE',  ( 0.000000000000000000, 0.000000000000000000, 1.000000000000000000 ) ) ;
#15407=CARTESIAN_POINT ( 'NONE',  ( -4.499999999708154341, 35.49999999900384751, -19.50000000000000355 ) ) ;
#15425=EDGE_LOOP ( 'NONE', ( #2771, #12648, #17823, #20709 ) ) ;
#15427=ORIENTED_EDGE ( 'NONE', *, *, #10356, .T. ) ;
#15434=CARTESIAN_POINT ( 'NONE',  ( 0.4500000002918510544, 42.99999999900385461, -19.00000000000000355 ) ) ;
#15438=DIRECTION ( 'NONE',  ( -1.000000000000000000, 0.000000000000000000, 0.000000000000000000 ) ) ;
#15449=ORIENTED_EDGE ( 'NONE', *, *, #2788, .T. ) ;
#15450=EDGE_LOOP ( 'NONE', ( #14737, #22851 ) ) ;
#15473=CARTESIAN_POINT ( 'NONE',  ( 2.918498775983380256E-10, 2.999999999003851503, -5.999999999999998224 ) ) ;
#15477=FACE_OUTER_BOUND ( 'NONE', #8759, .T. ) ;
#15491=PLANE ( 'NONE',  #1747 ) ;
#15499=ADVANCED_FACE ( 'NONE', ( #9776 ), #6022, .T. ) ;
#15505=CARTESIAN_POINT ( 'NONE',  ( -5.197224361976157780, 35.99999999900384751, -25.50000000000000000 ) ) ;
#15523=DIRECTION ( 'NONE',  ( 0.000000000000000000, -1.000000000000000000, 0.000000000000000000 ) ) ;
#15532=LINE ( 'NONE', #1765, #12667 ) ;
#15565=FACE_OUTER_BOUND ( 'NONE', #14487, .T. ) ;
#15566=EDGE_CURVE ( 'NONE', #10116, #145, #8781, .T. ) ;
#15579=DIRECTION ( 'NONE',  ( -0.000000000000000000, -0.000000000000000000, 1.000000000000000000 ) ) ;
#15586=CARTESIAN_POINT ( 'NONE',  ( -3.999999999708139686, 13.32455531934060744, -29.00000000000000355 ) ) ;
#15598=DIRECTION ( 'NONE',  ( 0.000000000000000000, 0.000000000000000000, 1.000000000000000000 ) ) ;
#15600=DIRECTION ( 'NONE',  ( 0.7071067811865474617, -0.7071067811865474617, 0.000000000000000000 ) ) ;
#15601=ORIENTED_EDGE ( 'NONE', *, *, #4648, .T. ) ;
#15602=EDGE_LOOP ( 'NONE', ( #18913, #20488, #9369, #20559 ) ) ;
#15603=ORIENTED_EDGE ( 'NONE', *, *, #18305, .T. ) ;
#15605=CARTESIAN_POINT ( 'NONE',  ( -3.999999999708153453, 42.99999999900385461, -29.00000000000000355 ) ) ;
#15612=CARTESIAN_POINT ( 'NONE',  ( -4.550510256924974684, 35.99999999900384751, -19.50000000000000355 ) ) ;
#15617=DIRECTION ( 'NONE',  ( -0.000000000000000000, 1.000000000000000000, -0.000000000000000000 ) ) ;
#15619=CARTESIAN_POINT ( 'NONE',  ( 30.00000000029184832, -9.961476088449217059E-10, -5.999999999999998224 ) ) ;
#15620=DIRECTION ( 'NONE',  ( -0.7071067811865492381, -0.7071067811865457964, 0.000000000000000000 ) ) ;
#15626=EDGE_CURVE ( 'NONE', #17223, #2802, #22237, .T. ) ;
#15631=ORIENTED_EDGE ( 'NONE', *, *, #19750, .T. ) ;
#15645=DIRECTION ( 'NONE',  ( -1.000000000000000000, 0.000000000000000000, 0.000000000000000000 ) ) ;
#15655=VERTEX_POINT ( 'NONE', #7860 ) ;
#15658=CARTESIAN_POINT ( 'NONE',  ( 2.918498775983380256E-10, -9.961476088449217059E-10, -19.00000000000000355 ) ) ;
#15667=DIRECTION ( 'NONE',  ( -0.000000000000000000, -0.000000000000000000, 1.000000000000000000 ) ) ;
#15675=ORIENTED_EDGE ( 'NONE', *, *, #4798, .T. ) ;
#15686=DIRECTION ( 'NONE',  ( 1.000000000000000000, 0.000000000000000000, 0.000000000000000000 ) ) ;
#15691=DIRECTION ( 'NONE',  ( -0.000000000000000000, -0.000000000000000000, 1.000000000000000000 ) ) ;
#15701=FACE_BOUND ( 'NONE', #18621, .T. ) ;
#15702=CARTESIAN_POINT ( 'NONE',  ( -6.899936419963482059, 13.99939863585067990, -18.20594370724277056 ) ) ;
#15704=DIRECTION ( 'NONE',  ( 0.000000000000000000, 1.000000000000000000, 0.000000000000000000 ) ) ;
#15713=VECTOR ( 'NONE', #4153, 1000.000000000000000 ) ;
#15715=ORIENTED_EDGE ( 'NONE', *, *, #22752, .T. ) ;
#15723=ADVANCED_FACE ( 'NONE', ( #6984 ), #19322, .F. ) ;
#15733=LINE ( 'NONE', #3621, #16708 ) ;
#15759=DIRECTION ( 'NONE',  ( -0.7071067811865475727, -0.7071067811865475727, 0.000000000000000000 ) ) ;
#15769=ORIENTED_EDGE ( 'NONE', *, *, #3475, .T. ) ;
#15799=CYLINDRICAL_SURFACE ( 'NONE', #20849, 2.550000000000002043 ) ;
#15806=CIRCLE ( 'NONE', #8691, 2.550000000000000266 ) ;
#15820=EDGE_CURVE ( 'NONE', #2725, #19136, #11328, .T. ) ;
#15833=DIRECTION ( 'NONE',  ( -1.000000000000000000, 0.000000000000000000, 0.000000000000000000 ) ) ;
#15836=CARTESIAN_POINT ( 'NONE',  ( 2.918498775983380256E-10, -9.961476088449217059E-10, 0.000000000000000000 ) ) ;
#15838=LINE ( 'NONE', #19380, #8162 ) ;
#15850=CARTESIAN_POINT ( 'NONE',  ( -5.423466998235942249, 35.99999999900384751, -25.65320998347783288 ) ) ;
#15861=DIRECTION ( 'NONE',  ( 0.7071067811865474617, -0.7071067811865474617, 0.000000000000000000 ) ) ;
#15884=CARTESIAN_POINT ( 'NONE',  ( -6.219322015043643681, 35.99999999900386172, -26.00774760879520642 ) ) ;
#15891=LINE ( 'NONE', #23104, #17663 ) ;
#15907=ORIENTED_EDGE ( 'NONE', *, *, #9880, .F. ) ;
#15913=ORIENTED_EDGE ( 'NONE', *, *, #14247, .T. ) ;
#15924=B_SPLINE_CURVE_WITH_KNOTS ( 'NONE', 3,
 ( #12294, #3382, #10541, #13349, #11454, #17322, #20531, #4276, #9937, #20648, #22634, #6293, #17088, #2991, #11570, #10161, #6409, #18756 ),
 .UNSPECIFIED., .F., .F.,
 ( 4, 2, 2, 2, 2, 2, 2, 2, 4 ),
 ( 0.000000000000000000, 0.0005979442104825547725, 0.001195888420965109545, 0.001793832631447664317, 0.002391776841930219090, 0.002989721052412773646, 0.003587665262895328635, 0.004185609473377883624, 0.004783553683860438180 ),
 .UNSPECIFIED. ) ;
#15954=DIRECTION ( 'NONE',  ( 1.000000000000000000, 0.000000000000000000, 0.000000000000000000 ) ) ;
#15993=PRESENTATION_STYLE_ASSIGNMENT (( #3317 ) ) ;
#15996=EDGE_CURVE ( 'NONE', #18159, #22993, #6106, .T. ) ;
#16006=CARTESIAN_POINT ( 'NONE',  ( -4.773379239211062774, 35.99999999900384751, -25.50000000000000355 ) ) ;
#16009=DIRECTION ( 'NONE',  ( -1.000000000000000000, 0.000000000000000000, 0.000000000000000000 ) ) ;
#16010=EDGE_CURVE ( 'NONE', #2292, #4567, #6468, .T. ) ;
#16029=EDGE_LOOP ( 'NONE', ( #14390, #12918, #1181, #1354 ) ) ;
#16036=VECTOR ( 'NONE', #11649, 1000.000000000000000 ) ;
#16043=CARTESIAN_POINT ( 'NONE',  ( 36.00000000029184832, 2.999999999003851503, 0.000000000000000000 ) ) ;
#16044=DIRECTION ( 'NONE',  ( 1.000000000000000000, 0.000000000000000000, 0.000000000000000000 ) ) ;
#16045=CARTESIAN_POINT ( 'NONE',  ( 6.000000000291855429, 2.999999999003851503, -39.00000000000000000 ) ) ;
#16047=CARTESIAN_POINT ( 'NONE',  ( -6.359599319592075695, 13.97158350606811617, -17.13641408681294109 ) ) ;
#16050=TOROIDAL_SURFACE ( 'NONE', #2151, 3.500000000000000000, 0.5000000000000000000 ) ;
#16072=DIRECTION ( 'NONE',  ( 0.000000000000000000, -1.000000000000000000, 0.000000000000000000 ) ) ;
#16082=CARTESIAN_POINT ( 'NONE',  ( 30.00000000029184832, 2.999999999003851503, 0.000000000000000000 ) ) ;
#16084=ORIENTED_EDGE ( 'NONE', *, *, #15566, .T. ) ;
#16097=CARTESIAN_POINT ( 'NONE',  ( 27.94974746859769255, 27.94974746730969528, -19.49999999999998934 ) ) ;
#16111=EDGE_CURVE ( 'NONE', #8379, #14963, #13854, .T. ) ;
#16112=ORIENTED_EDGE ( 'NONE', *, *, #7643, .F. ) ;
#16116=EDGE_LOOP ( 'NONE', ( #2467, #3429, #5729, #9886 ) ) ;
#16120=CARTESIAN_POINT ( 'NONE',  ( -4.550510256924974684, 36.49999999900384751, -25.50000000000000000 ) ) ;
#16122=CARTESIAN_POINT ( 'NONE',  ( 35.50000000029184832, 16.99999999900385461, -26.50000000000000000 ) ) ;
#16123=CARTESIAN_POINT ( 'NONE',  ( -6.962001439796694058, 35.99999999900384751, -18.52402997057235723 ) ) ;
#16134=CARTESIAN_POINT ( 'NONE',  ( 31.55000000029185259, 16.99999999900385461, -25.50000000000000355 ) ) ;
#16136=CARTESIAN_POINT ( 'NONE',  ( 2.918498775983380256E-10, 2.999999999003851503, 0.000000000000000000 ) ) ;
#16198=ORIENTED_EDGE ( 'NONE', *, *, #12498, .F. ) ;
#16199=CARTESIAN_POINT ( 'NONE',  ( -3.999999999708154341, 38.75225147438560924, -29.00000000000001066 ) ) ;
#16223=ORIENTED_EDGE ( 'NONE', *, *, #204, .T. ) ;
#16244=DIRECTION ( 'NONE',  ( 0.000000000000000000, 0.000000000000000000, -1.000000000000000000 ) ) ;
#16249=DIRECTION ( 'NONE',  ( -0.000000000000000000, -0.000000000000000000, 1.000000000000000000 ) ) ;
#16257=EDGE_CURVE ( 'NONE', #19696, #16772, #9604, .T. ) ;
#16260=ORIENTED_EDGE ( 'NONE', *, *, #20460, .F. ) ;
#16311=DIRECTION ( 'NONE',  ( 0.000000000000000000, -1.000000000000000000, 0.000000000000000000 ) ) ;
#16313=CARTESIAN_POINT ( 'NONE',  ( -3.999999999708153453, 38.99999999900385461, -18.50000000000000355 ) ) ;
#16327=DIRECTION ( 'NONE',  ( 0.000000000000000000, 0.000000000000000000, 1.000000000000000000 ) ) ;
#16335=CYLINDRICAL_SURFACE ( 'NONE', #1537, 5.999999999999998224 ) ;
#16337=CARTESIAN_POINT ( 'NONE',  ( -6.960550854630949580, 36.00005224601497389, -18.51506780978411015 ) ) ;
#16347=ORIENTED_EDGE ( 'NONE', *, *, #15820, .F. ) ;
#16349=ORIENTED_EDGE ( 'NONE', *, *, #22938, .T. ) ;
#16355=CARTESIAN_POINT ( 'NONE',  ( -3.999999999708139686, 35.99999999900384751, -18.99999999999998934 ) ) ;
#16358=CARTESIAN_POINT ( 'NONE',  ( -3.999999999708152121, 38.75225147438559503, -15.99999999999998579 ) ) ;
#16360=PLANE ( 'NONE',  #5777 ) ;
#16361=DIRECTION ( 'NONE',  ( 0.7071067811865474617, -0.7071067811865474617, 0.000000000000000000 ) ) ;
#16370=AXIS2_PLACEMENT_3D ( 'NONE', #13867, #22354, #17380 ) ;
#16376=ORIENTED_EDGE ( 'NONE', *, *, #7761, .F. ) ;
#16395=EDGE_CURVE ( 'NONE', #22474, #19191, #13613, .T. ) ;
#16397=EDGE_LOOP ( 'NONE', ( #13128, #199 ) ) ;
#16406=CYLINDRICAL_SURFACE ( 'NONE', #21200, 6.000000000000000000 ) ;
#16431=VECTOR ( 'NONE', #9382, 1000.000000000000000 ) ;
#16434=CARTESIAN_POINT ( 'NONE',  ( -5.122455540400329355, 36.64919863988808402, -28.78988827279798812 ) ) ;
#16445=AXIS2_PLACEMENT_3D ( 'NONE', #20240, #18934, #15620 ) ;
#16447=DIRECTION ( 'NONE',  ( 0.000000000000000000, 0.000000000000000000, 1.000000000000000000 ) ) ;
#16461=TOROIDAL_SURFACE ( 'NONE', #13102, 3.500000000000000000, 0.5000000000000000000 ) ;
#16480=DIRECTION ( 'NONE',  ( -0.000000000000000000, -1.000000000000000000, -0.000000000000000000 ) ) ;
#16488=ORIENTED_EDGE ( 'NONE', *, *, #19202, .F. ) ;
#16505=LINE ( 'NONE', #21945, #18938 ) ;
#16516=ORIENTED_EDGE ( 'NONE', *, *, #974, .F. ) ;
#16519=DIRECTION ( 'NONE',  ( -0.000000000000000000, 1.000000000000000000, -0.000000000000000000 ) ) ;
#16540=CARTESIAN_POINT ( 'NONE',  ( -4.938244945965067245, 36.80742465210829550, -28.85443706880898418 ) ) ;
#16557=ADVANCED_FACE ( 'NONE', ( #5359 ), #10754, .T. ) ;
#16563=SHAPE_DEFINITION_REPRESENTATION ( #19646, #10586 ) ;
#16578=CARTESIAN_POINT ( 'NONE',  ( 6.000000000291855429, -9.961476088449217059E-10, -5.999999999999998224 ) ) ;
#16586=CARTESIAN_POINT ( 'NONE',  ( 36.00000000029184832, -9.961476088449217059E-10, -5.999999999999998224 ) ) ;
#16600=AXIS2_PLACEMENT_3D ( 'NONE', #6743, #8509, #22751 ) ;
#16611=EDGE_CURVE ( 'NONE', #13097, #555, #22646, .T. ) ;
#16612=AXIS2_PLACEMENT_3D ( 'NONE', #8282, #2632, #18630 ) ;
#16615=DIRECTION ( 'NONE',  ( 0.000000000000000000, 0.000000000000000000, 1.000000000000000000 ) ) ;
#16619=EDGE_CURVE ( 'NONE', #19937, #19243, #2713, .T. ) ;
#16629=VERTEX_POINT ( 'NONE', #22277 ) ;
#16661=AXIS2_PLACEMENT_3D ( 'NONE', #20174, #8045, #14983 ) ;
#16668=CARTESIAN_POINT ( 'NONE',  ( 5.550000000291854363, 42.99999999900385461, -26.00000000000000000 ) ) ;
#16682=( GEOMETRIC_REPRESENTATION_CONTEXT ( 3 ) GLOBAL_UNCERTAINTY_ASSIGNED_CONTEXT ( ( #5818 ) ) GLOBAL_UNIT_ASSIGNED_CONTEXT ( ( #4146, #22618, #9800 ) ) REPRESENTATION_CONTEXT ( 'NONE', 'WORKASPACE' ) );
#16695=CARTESIAN_POINT ( 'NONE',  ( 3.000000000291852764, 42.99999999900385461, 0.000000000000000000 ) ) ;
#16707=EDGE_CURVE ( 'NONE', #371, #3970, #4984, .T. ) ;
#16708=VECTOR ( 'NONE', #17496, 1000.000000000000000 ) ;
#16710=LINE ( 'NONE', #7250, #21211 ) ;
#16713=CARTESIAN_POINT ( 'NONE',  ( 6.000000000291855429, -9.961476088449217059E-10, -39.00000000000000000 ) ) ;
#16714=ORIENTED_EDGE ( 'NONE', *, *, #17872, .T. ) ;
#16739=DIRECTION ( 'NONE',  ( -1.000000000000000000, -0.000000000000000000, 0.000000000000000000 ) ) ;
#16743=DIRECTION ( 'NONE',  ( 0.000000000000000000, 0.000000000000000000, 1.000000000000000000 ) ) ;
#16744=VERTEX_POINT ( 'NONE', #21095 ) ;
#16746=ORIENTED_EDGE ( 'NONE', *, *, #17269, .F. ) ;
#16748=AXIS2_PLACEMENT_3D ( 'NONE', #18676, #9170, #16327 ) ;
#16754=LINE ( 'NONE', #666, #14400 ) ;
#16772=VERTEX_POINT ( 'NONE', #3220 ) ;
#16776=CARTESIAN_POINT ( 'NONE',  ( -4.550510256924974684, 36.49999999900384751, -19.00000000000000355 ) ) ;
#16787=DIRECTION ( 'NONE',  ( 1.000000000000000000, 0.000000000000000000, 0.000000000000000000 ) ) ;
#16791=AXIS2_PLACEMENT_3D ( 'NONE', #12877, #9236, #20061 ) ;
#16795=VECTOR ( 'NONE', #16249, 1000.000000000000000 ) ;
#16806=LINE ( 'NONE', #22243, #10478 ) ;
#16811=CARTESIAN_POINT ( 'NONE',  ( -4.614318463248863189, 37.16513102274243607, -16.05878810958467895 ) ) ;
#16814=DIRECTION ( 'NONE',  ( 0.000000000000000000, 0.000000000000000000, 1.000000000000000000 ) ) ;
#16815=DIRECTION ( 'NONE',  ( -0.000000000000000000, -0.000000000000000000, 1.000000000000000000 ) ) ;
#16819=CARTESIAN_POINT ( 'NONE',  ( 29.00000000029184832, 16.99999999900385461, -19.00000000000000355 ) ) ;
#16823=ADVANCED_FACE ( 'NONE', ( #22513 ), #17434, .T. ) ;
#16825=CARTESIAN_POINT ( 'NONE',  ( 6.000000000291855429, 2.999999999003851503, 0.000000000000000000 ) ) ;
#16832=EDGE_LOOP ( 'NONE', ( #9215, #18877, #20329, #11894 ) ) ;
#16838=CARTESIAN_POINT ( 'NONE',  ( 2.918498775983380256E-10, -9.961476088449217059E-10, -5.999999999999998224 ) ) ;
#16846=CIRCLE ( 'NONE', #4833, 1.000000000000000000 ) ;
#16851=FACE_OUTER_BOUND ( 'NONE', #1541, .T. ) ;
#16865=VERTEX_POINT ( 'NONE', #19910 ) ;
#16873=EDGE_CURVE ( 'NONE', #9093, #4926, #12482, .T. ) ;
#16878=DIRECTION ( 'NONE',  ( -0.000000000000000000, -0.000000000000000000, 1.000000000000000000 ) ) ;
#16887=LINE ( 'NONE', #2664, #15261 ) ;
#16903=EDGE_CURVE ( 'NONE', #5703, #8151, #1993, .T. ) ;
#16904=CARTESIAN_POINT ( 'NONE',  ( -6.979889398549481427, 35.99999999900384751, -18.51271870087857607 ) ) ;
#16922=CARTESIAN_POINT ( 'NONE',  ( -6.999999999708142795, 38.99999999900385461, -22.50000000000000000 ) ) ;
#16928=DIRECTION ( 'NONE',  ( 0.000000000000000000, 0.000000000000000000, -1.000000000000000000 ) ) ;
#16929=CARTESIAN_POINT ( 'NONE',  ( -4.499999999708154341, 35.99999999900384751, -19.50000000000000355 ) ) ;
#16942=ORIENTED_EDGE ( 'NONE', *, *, #19160, .F. ) ;
#16946=ORIENTED_EDGE ( 'NONE', *, *, #11153, .F. ) ;
#16968=DIRECTION ( 'NONE',  ( 0.000000000000000000, 0.000000000000000000, -1.000000000000000000 ) ) ;
#16976=ORIENTED_EDGE ( 'NONE', *, *, #7575, .F. ) ;
#16994=LINE ( 'NONE', #15473, #8792 ) ;
#16997=CIRCLE ( 'NONE', #20778, 7.000000000000000000 ) ;
#17003=CARTESIAN_POINT ( 'NONE',  ( -3.999999999708139686, 49.99999999900385461, -26.00000000000000711 ) ) ;
#17012=CIRCLE ( 'NONE', #514, 7.000000000000000000 ) ;
#17034=LINE ( 'NONE', #20834, #4813 ) ;
#17050=FACE_OUTER_BOUND ( 'NONE', #15200, .T. ) ;
#17055=CARTESIAN_POINT ( 'NONE',  ( 36.00000000029184832, 5.999999999003851059, -12.99999999999999822 ) ) ;
#17064=CIRCLE ( 'NONE', #21615, 0.5000000000000004441 ) ;
#17070=EDGE_LOOP ( 'NONE', ( #5293, #21667, #13327, #5582, #15769 ) ) ;
#17082=CARTESIAN_POINT ( 'NONE',  ( 5.550000000291854363, 42.99999999900385461, -29.00000000000000355 ) ) ;
#17088=CARTESIAN_POINT ( 'NONE',  ( -6.683546854663851455, 13.99327871316343952, -27.35588422962999999 ) ) ;
#17094=ORIENTED_EDGE ( 'NONE', *, *, #23064, .F. ) ;
#17102=ORIENTED_EDGE ( 'NONE', *, *, #3459, .T. ) ;
#17109=FACE_OUTER_BOUND ( 'NONE', #17215, .T. ) ;
#17115=DIRECTION ( 'NONE',  ( -0.000000000000000000, -0.000000000000000000, -1.000000000000000000 ) ) ;
#17127=ORIENTED_EDGE ( 'NONE', *, *, #5574, .F. ) ;
#17152=EDGE_CURVE ( 'NONE', #5983, #20043, #13425, .T. ) ;
#17163=VECTOR ( 'NONE', #8687, 1000.000000000000000 ) ;
#17173=CARTESIAN_POINT ( 'NONE',  ( 35.50000000029184832, -9.961476088449217059E-10, -19.00000000000000355 ) ) ;
#17180=CARTESIAN_POINT ( 'NONE',  ( 33.59619407800440882, 21.59619407671641866, -18.50000000000000355 ) ) ;
#17181=EDGE_CURVE ( 'NONE', #9160, #5703, #9893, .T. ) ;
#17197=CIRCLE ( 'NONE', #5952, 0.4999999999999994449 ) ;
#17215=EDGE_LOOP ( 'NONE', ( #2241, #20426, #22559, #3600 ) ) ;
#17219=ORIENTED_EDGE ( 'NONE', *, *, #22981, .T. ) ;
#17223=VERTEX_POINT ( 'NONE', #16929 ) ;
#17224=DIRECTION ( 'NONE',  ( 0.000000000000000000, 0.000000000000000000, 1.000000000000000000 ) ) ;
#17227=CARTESIAN_POINT ( 'NONE',  ( 6.000000000291855429, 2.999999999003851503, -39.00000000000000000 ) ) ;
#17233=DIRECTION ( 'NONE',  ( -1.000000000000000000, 0.000000000000000000, 1.613696256722611405E-16 ) ) ;
#17254=ADVANCED_FACE ( 'NONE', ( #11993 ), #12884, .T. ) ;
#17257=AXIS2_PLACEMENT_3D ( 'NONE', #17227, #1137, #13715 ) ;
#17268=ORIENTED_EDGE ( 'NONE', *, *, #1681, .T. ) ;
#17269=EDGE_CURVE ( 'NONE', #5235, #9785, #17285, .T. ) ;
#17273=EDGE_CURVE ( 'NONE', #343, #2319, #135, .T. ) ;
#17285=LINE ( 'NONE', #22719, #4232 ) ;
#17292=( LENGTH_UNIT ( ) NAMED_UNIT ( * ) SI_UNIT ( .MILLI., .METRE. ) );
#17295=ADVANCED_FACE ( 'NONE', ( #6831 ), #4935, .F. ) ;
#17319=LINE ( 'NONE', #17558, #13064 ) ;
#17322=CARTESIAN_POINT ( 'NONE',  ( -5.281014309470088541, 13.78823385074812613, -28.71965152573269719 ) ) ;
#17331=EDGE_CURVE ( 'NONE', #14653, #5722, #8709, .T. ) ;
#17343=CARTESIAN_POINT ( 'NONE',  ( 29.00000000029184832, 16.99999999900385461, -19.49999999999998934 ) ) ;
#17354=DIRECTION ( 'NONE',  ( 0.000000000000000000, -1.000000000000000000, 0.000000000000000000 ) ) ;
#17380=DIRECTION ( 'NONE',  ( 1.000000000000000000, 0.000000000000000000, -0.000000000000000000 ) ) ;
#17382=DIRECTION ( 'NONE',  ( -0.000000000000000000, -1.000000000000000000, 0.000000000000000000 ) ) ;
#17395=CARTESIAN_POINT ( 'NONE',  ( -4.950765356264206218, 36.36782871084107427, -26.02439111740734035 ) ) ;
#17401=EDGE_CURVE ( 'NONE', #15368, #14653, #5021, .T. ) ;
#17405=DIRECTION ( 'NONE',  ( 1.000000000000000000, 0.000000000000000000, 0.000000000000000000 ) ) ;
#17409=CARTESIAN_POINT ( 'NONE',  ( -6.958039891257955745, 36.00029345514013102, -18.49999999999999645 ) ) ;
#17415=EDGE_CURVE ( 'NONE', #3554, #20913, #9162, .T. ) ;
#17419=EDGE_CURVE ( 'NONE', #8586, #14201, #5650, .T. ) ;
#17420=EDGE_LOOP ( 'NONE', ( #2378, #11580, #18276, #7128 ) ) ;
#17421=VECTOR ( 'NONE', #3478, 1000.000000000000000 ) ;
#17434=CYLINDRICAL_SURFACE ( 'NONE', #20001, 5.999999999999998224 ) ;
#17447=EDGE_CURVE ( 'NONE', #690, #13411, #22311, .T. ) ;
#17452=ORIENTED_EDGE ( 'NONE', *, *, #23064, .T. ) ;
#17453=ORIENTED_EDGE ( 'NONE', *, *, #15626, .T. ) ;
#17464=CARTESIAN_POINT ( 'NONE',  ( 3.000000000291852764, 42.99999999900385461, -19.49999999999998934 ) ) ;
#17472=CARTESIAN_POINT ( 'NONE',  ( -6.587771436282949367, 13.98878796535109359, -17.46895447544054747 ) ) ;
#17479=DIRECTION ( 'NONE',  ( 0.000000000000000000, 0.000000000000000000, 1.000000000000000000 ) ) ;
#17482=EDGE_CURVE ( 'NONE', #8658, #343, #14024, .T. ) ;
#17484=ORIENTED_EDGE ( 'NONE', *, *, #13980, .T. ) ;
#17496=DIRECTION ( 'NONE',  ( -0.000000000000000000, -0.000000000000000000, 1.000000000000000000 ) ) ;
#17522=DIRECTION ( 'NONE',  ( -0.000000000000000000, 1.000000000000000000, -0.000000000000000000 ) ) ;
#17536=EDGE_CURVE ( 'NONE', #4283, #22262, #9528, .T. ) ;
#17545=AXIS2_PLACEMENT_3D ( 'NONE', #8458, #20700, #4803 ) ;
#17558=CARTESIAN_POINT ( 'NONE',  ( -3.499999999708153453, 35.99999999900384751, -19.00000000000000355 ) ) ;
#17572=AXIS2_PLACEMENT_3D ( 'NONE', #5877, #18680, #3863 ) ;
#17581=CARTESIAN_POINT ( 'NONE',  ( -6.999999999708156118, 6.999999999003851947, -19.00000000000000355 ) ) ;
#17595=EDGE_LOOP ( 'NONE', ( #8664, #2647, #23129, #2379, #8516, #12266, #8213, #10166, #15135, #7172, #3026, #22615, #65 ) ) ;
#17598=CARTESIAN_POINT ( 'NONE',  ( 26.09619407800441948, 29.09619407671641866, -26.00000000000000000 ) ) ;
#17602=ORIENTED_EDGE ( 'NONE', *, *, #14532, .F. ) ;
#17605=ORIENTED_EDGE ( 'NONE', *, *, #3258, .T. ) ;
#17629=FACE_OUTER_BOUND ( 'NONE', #19129, .T. ) ;
#17637=CARTESIAN_POINT ( 'NONE',  ( -5.197224361976157780, 36.49999999900384751, -19.00000000000000355 ) ) ;
#17649=( LENGTH_UNIT ( ) NAMED_UNIT ( * ) SI_UNIT ( .MILLI., .METRE. ) );
#17663=VECTOR ( 'NONE', #23218, 1000.000000000000000 ) ;
#17673=LINE ( 'NONE', #5222, #10797 ) ;
#17689=CYLINDRICAL_SURFACE ( 'NONE', #18205, 7.000000000000006217 ) ;
#17706=CARTESIAN_POINT ( 'NONE',  ( 30.00000000029184832, -0.5000000009961480529, -39.00000000000000000 ) ) ;
#17714=ORIENTED_EDGE ( 'NONE', *, *, #22576, .F. ) ;
#17729=CARTESIAN_POINT ( 'NONE',  ( -3.499999999708153453, 13.99999999900385106, -19.50000000000000355 ) ) ;
#17731=EDGE_CURVE ( 'NONE', #16744, #10365, #14779, .T. ) ;
#17737=CARTESIAN_POINT ( 'NONE',  ( 2.918498775983380256E-10, 2.999999999003851503, -39.00000000000000000 ) ) ;
#17740=CIRCLE ( 'NONE', #7985, 2.550000000000000711 ) ;
#17743=ORIENTED_EDGE ( 'NONE', *, *, #3231, .F. ) ;
#17752=AXIS2_PLACEMENT_3D ( 'NONE', #21598, #14517, #21707 ) ;
#17763=FACE_OUTER_BOUND ( 'NONE', #6564, .T. ) ;
#17766=CARTESIAN_POINT ( 'NONE',  ( -3.999999999708153453, 35.49999999900384751, -19.50000000000000355 ) ) ;
#17774=( NAMED_UNIT ( * ) SI_UNIT ( $, .STERADIAN. ) SOLID_ANGLE_UNIT ( ) );
#17784=EDGE_CURVE ( 'NONE', #12152, #12647, #7926, .T. ) ;
#17788=ORIENTED_EDGE ( 'NONE', *, *, #19, .T. ) ;
#17816=EDGE_LOOP ( 'NONE', ( #16223, #5336, #7182, #1009 ) ) ;
#17823=ORIENTED_EDGE ( 'NONE', *, *, #32, .F. ) ;
#17824=CARTESIAN_POINT ( 'NONE',  ( -3.499999999708153453, 2.999999999003851503, -26.00000000000000000 ) ) ;
#17834=VECTOR ( 'NONE', #16519, 1000.000000000000000 ) ;
#17844=ORIENTED_EDGE ( 'NONE', *, *, #3475, .F. ) ;
#17849=ADVANCED_FACE ( 'NONE', ( #6175 ), #2164, .T. ) ;
#17857=DIRECTION ( 'NONE',  ( 0.000000000000000000, 0.000000000000000000, 1.000000000000000000 ) ) ;
#17863=EDGE_CURVE ( 'NONE', #19813, #14653, #16505, .T. ) ;
#17869=LINE ( 'NONE', #16082, #14931 ) ;
#17870=EDGE_LOOP ( 'NONE', ( #12092, #10467 ) ) ;
#17872=EDGE_CURVE ( 'NONE', #14621, #10396, #21215, .T. ) ;
#17873=CARTESIAN_POINT ( 'NONE',  ( -6.977878452269129284, 35.99999999900352776, -26.49046115436484783 ) ) ;
#17879=ORIENTED_EDGE ( 'NONE', *, *, #3494, .F. ) ;
#17895=AXIS2_PLACEMENT_3D ( 'NONE', #21968, #16311, #11015 ) ;
#17900=EDGE_LOOP ( 'NONE', ( #6731, #17903 ) ) ;
#17903=ORIENTED_EDGE ( 'NONE', *, *, #13983, .T. ) ;
#17904=ORIENTED_EDGE ( 'NONE', *, *, #10404, .F. ) ;
#17932=EDGE_LOOP ( 'NONE', ( #17879, #146, #7661, #8470, #9136, #9223, #1267, #9331, #12654, #11606, #8609, #1811, #22152 ) ) ;
#17952=CARTESIAN_POINT ( 'NONE',  ( -4.920724633012840243, 13.68667664578917709, -16.13822288903187996 ) ) ;
#17958=LINE ( 'NONE', #5372, #7859 ) ;
#17967=ORIENTED_EDGE ( 'NONE', *, *, #5831, .F. ) ;
#17974=DIRECTION ( 'NONE',  ( 0.000000000000000000, -1.000000000000000000, 0.000000000000000000 ) ) ;
#17979=AXIS2_PLACEMENT_3D ( 'NONE', #3074, #8486, #15645 ) ;
#17981=VECTOR ( 'NONE', #3313, 1000.000000000000000 ) ;
#17982=AXIS2_PLACEMENT_3D ( 'NONE', #13829, #11829, #19232 ) ;
#17984=LINE ( 'NONE', #21637, #17163 ) ;
#17993=CARTESIAN_POINT ( 'NONE',  ( -5.498446330623528056, 36.40058408549441538, -28.60140285650649972 ) ) ;
#18037=EDGE_CURVE ( 'NONE', #13010, #3689, #263, .T. ) ;
#18044=CARTESIAN_POINT ( 'NONE',  ( 2.918498775983380256E-10, -9.961476088449217059E-10, 0.000000000000000000 ) ) ;
#18056=ORIENTED_EDGE ( 'NONE', *, *, #19611, .F. ) ;
#18076=VERTEX_POINT ( 'NONE', #14613 ) ;
#18081=CIRCLE ( 'NONE', #3793, 0.5000000000000004441 ) ;
#18090=DIRECTION ( 'NONE',  ( 1.000000000000000000, 0.000000000000000000, 0.000000000000000000 ) ) ;
#18102=CARTESIAN_POINT ( 'NONE',  ( -6.549842551561727788, 36.00336057837472481, -18.61861813964035761 ) ) ;
#18110=CARTESIAN_POINT ( 'NONE',  ( -3.499999999708153453, 38.99999999900385461, -19.00000000000000355 ) ) ;
#18136=DIRECTION ( 'NONE',  ( 0.000000000000000000, 1.000000000000000000, 0.000000000000000000 ) ) ;
#18156=ORIENTED_EDGE ( 'NONE', *, *, #22185, .T. ) ;
#18159=VERTEX_POINT ( 'NONE', #9778 ) ;
#18181=CARTESIAN_POINT ( 'NONE',  ( 30.00000000029184832, -0.5000000009961480529, -41.54999999999999716 ) ) ;
#18189=DIRECTION ( 'NONE',  ( 1.000000000000000000, 0.000000000000000000, 0.000000000000000000 ) ) ;
#18198=EDGE_LOOP ( 'NONE', ( #8058, #15345, #17602, #12041 ) ) ;
#18199=ORIENTED_EDGE ( 'NONE', *, *, #2887, .F. ) ;
#18205=AXIS2_PLACEMENT_3D ( 'NONE', #3465, #15579, #21365 ) ;
#18212=LINE ( 'NONE', #328, #16431 ) ;
#18221=CARTESIAN_POINT ( 'NONE',  ( -6.958039891257955745, 36.00029345514013102, -26.50000000000000000 ) ) ;
#18224=CARTESIAN_POINT ( 'NONE',  ( -5.350349885510485848, 36.24720445779466615, -18.90862932150717413 ) ) ;
#18228=CARTESIAN_POINT ( 'NONE',  ( 36.00000000029184832, 2.999999999003851503, -39.00000000000000000 ) ) ;
#18230=DIRECTION ( 'NONE',  ( 1.000000000000000000, 0.000000000000000000, 0.000000000000000000 ) ) ;
#18233=CARTESIAN_POINT ( 'NONE',  ( -6.999999999708142795, 38.99999999900385461, -18.50000000000000355 ) ) ;
#18237=DIRECTION ( 'NONE',  ( -0.000000000000000000, -0.000000000000000000, 1.000000000000000000 ) ) ;
#18243=EDGE_CURVE ( 'NONE', #14311, #2294, #10625, .T. ) ;
#18246=ORIENTED_EDGE ( 'NONE', *, *, #21101, .T. ) ;
#18247=EDGE_CURVE ( 'NONE', #12125, #16865, #496, .T. ) ;
#18254=CARTESIAN_POINT ( 'NONE',  ( -6.226186441994415510, 36.09747688189035841, -16.97411279881559310 ) ) ;
#18268=ORIENTED_EDGE ( 'NONE', *, *, #6153, .F. ) ;
#18276=ORIENTED_EDGE ( 'NONE', *, *, #5616, .F. ) ;
#18286=AXIS2_PLACEMENT_3D ( 'NONE', #12641, #16743, #2288 ) ;
#18305=EDGE_CURVE ( 'NONE', #8962, #888, #18950, .T. ) ;
#18314=CARTESIAN_POINT ( 'NONE',  ( 35.50000000029184832, -9.961476088449217059E-10, -26.50000000000000000 ) ) ;
#18323=VECTOR ( 'NONE', #19562, 1000.000000000000000 ) ;
#18372=LINE ( 'NONE', #11186, #20314 ) ;
#18435=ADVANCED_BREP_SHAPE_REPRESENTATION ( '', ( #12837, #22115 ), #7836 ) ;
#18437=CARTESIAN_POINT ( 'NONE',  ( 2.918498775983380256E-10, 6.999999999003851947, -19.00000000000000355 ) ) ;
#18442=CARTESIAN_POINT ( 'NONE',  ( 6.000000000291855429, 2.999999999003851503, -5.999999999999998224 ) ) ;
#18460=CARTESIAN_POINT ( 'NONE',  ( 3.000000000291852764, 42.99999999900385461, -26.50000000000000000 ) ) ;
#18474=CYLINDRICAL_SURFACE ( 'NONE', #1130, 6.999999999999999112 ) ;
#18488=AXIS2_PLACEMENT_3D ( 'NONE', #22691, #8216, #15833 ) ;
#18499=AXIS2_PLACEMENT_3D ( 'NONE', #2255, #16815, #615 ) ;
#18517=CYLINDRICAL_SURFACE ( 'NONE', #14820, 0.5000000000000000000 ) ;
#18545=VECTOR ( 'NONE', #14083, 1000.000000000000000 ) ;
#18557=CIRCLE ( 'NONE', #8427, 2.550000000000003819 ) ;
#18584=COLOUR_RGB ( '', 0.09019608, 0.27058824, 0.51372549) ;
#18604=CARTESIAN_POINT ( 'NONE',  ( -6.525612274168518745, 36.03379296756838812, -17.36249956737804112 ) ) ;
#18610=DIRECTION ( 'NONE',  ( 0.000000000000000000, 0.000000000000000000, -1.000000000000000000 ) ) ;
#18611=CARTESIAN_POINT ( 'NONE',  ( 0.4500000002918510544, 42.99999999900385461, -19.49999999999998934 ) ) ;
#18621=EDGE_LOOP ( 'NONE', ( #7481, #16714 ) ) ;
#18622=EDGE_CURVE ( 'NONE', #14963, #6361, #17012, .T. ) ;
#18630=DIRECTION ( 'NONE',  ( 0.000000000000000000, 0.000000000000000000, 1.000000000000000000 ) ) ;
#18647=CIRCLE ( 'NONE', #1010, 2.550000000000002043 ) ;
#18656=CARTESIAN_POINT ( 'NONE',  ( 31.55000000029185259, 16.99999999900385461, -15.99999999999999289 ) ) ;
#18658=DIRECTION ( 'NONE',  ( 0.000000000000000000, 0.000000000000000000, 1.000000000000000000 ) ) ;
#18659=CARTESIAN_POINT ( 'NONE',  ( -6.999999999708142795, 13.99999999900385106, -19.00000000000000355 ) ) ;
#18676=CARTESIAN_POINT ( 'NONE',  ( 30.00000000029184832, -9.961476088449217059E-10, -39.00000000000000000 ) ) ;
#18680=DIRECTION ( 'NONE',  ( -0.000000000000000000, -0.000000000000000000, 1.000000000000000000 ) ) ;
#18712=DIRECTION ( 'NONE',  ( 0.000000000000000000, 0.000000000000000000, -1.000000000000000000 ) ) ;
#18718=AXIS2_PLACEMENT_3D ( 'NONE', #7507, #20094, #569 ) ;
#18726=EDGE_CURVE ( 'NONE', #12296, #4090, #6896, .T. ) ;
#18731=ORIENTED_EDGE ( 'NONE', *, *, #21101, .F. ) ;
#18736=CARTESIAN_POINT ( 'NONE',  ( 6.000000000291855429, -0.5000000009961480529, -39.00000000000000000 ) ) ;
#18739=FILL_AREA_STYLE ('',( #9576 ) ) ;
#18743=DIRECTION ( 'NONE',  ( 0.000000000000000000, -1.000000000000000000, 0.000000000000000000 ) ) ;
#18744=LINE ( 'NONE', #6170, #13544 ) ;
#18756=CARTESIAN_POINT ( 'NONE',  ( -6.999999999708142795, 13.99999999900385106, -26.00000000000000000 ) ) ;
#18764=EDGE_LOOP ( 'NONE', ( #3973, #17743 ) ) ;
#18783=CARTESIAN_POINT ( 'NONE',  ( 2.918498775983380256E-10, 6.999999999003851947, -29.00000000000000355 ) ) ;
#18806=CARTESIAN_POINT ( 'NONE',  ( -4.993857080238742974, 35.99999999900384751, -19.46409504053740491 ) ) ;
#18821=CARTESIAN_POINT ( 'NONE',  ( 33.94974746859769255, 21.94974746730969528, -29.00000000000000355 ) ) ;
#18839=ORIENTED_EDGE ( 'NONE', *, *, #10404, .T. ) ;
#18850=ORIENTED_EDGE ( 'NONE', *, *, #15065, .F. ) ;
#18851=SURFACE_SIDE_STYLE ('',( #13212 ) ) ;
#18855=CARTESIAN_POINT ( 'NONE',  ( 2.918498775983380256E-10, -9.961476088449217059E-10, -39.00000000000000000 ) ) ;
#18860=AXIS2_PLACEMENT_3D ( 'NONE', #8095, #15255, #4094 ) ;
#18863=DIRECTION ( 'NONE',  ( -1.858632295689435609E-16, -1.000000000000000000, 0.000000000000000000 ) ) ;
#18877=ORIENTED_EDGE ( 'NONE', *, *, #20460, .T. ) ;
#18888=VERTEX_POINT ( 'NONE', #17737 ) ;
#18895=DIRECTION ( 'NONE',  ( 1.000000000000000000, 0.000000000000000000, 0.000000000000000000 ) ) ;
#18904=CARTESIAN_POINT ( 'NONE',  ( 27.94974746859769255, 27.94974746730969528, -18.50000000000000355 ) ) ;
#18906=EDGE_LOOP ( 'NONE', ( #13202, #1305, #15631, #17714 ) ) ;
#18909=FACE_OUTER_BOUND ( 'NONE', #18974, .T. ) ;
#18913=ORIENTED_EDGE ( 'NONE', *, *, #19750, .F. ) ;
#18923=PLANE ( 'NONE',  #21314 ) ;
#18926=CARTESIAN_POINT ( 'NONE',  ( -6.231825765915511184, 35.99999999900384751, -18.98541138272435802 ) ) ;
#18934=DIRECTION ( 'NONE',  ( -0.7071067811865457964, 0.7071067811865492381, 0.000000000000000000 ) ) ;
#18936=CIRCLE ( 'NONE', #151, 6.000000000000000000 ) ;
#18938=VECTOR ( 'NONE', #16739, 1000.000000000000000 ) ;
#18950=CIRCLE ( 'NONE', #21548, 2.550000000000002043 ) ;
#18957=CARTESIAN_POINT ( 'NONE',  ( -3.499999999708153453, 13.99999999900385106, -26.00000000000000000 ) ) ;
#18974=EDGE_LOOP ( 'NONE', ( #22031, #20943, #21832, #8750, #22953, #13598, #15715 ) ) ;
#18998=B_SPLINE_CURVE_WITH_KNOTS ( 'NONE', 3,
 ( #18221, #13035, #13157, #7623, #21860, #1858, #4191, #12920, #2087, #17993, #9043, #16434, #16540, #340, #20099, #3971, #20219, #11148, #16199, #14461 ),
 .UNSPECIFIED., .F., .F.,
 ( 4, 2, 2, 2, 2, 2, 2, 2, 2, 4 ),
 ( 0.0005000078514897923158, 0.001232179299099181967, 0.001964350746708571835, 0.002696522194317961703, 0.003062607918122655336, 0.003428693641927348969, 0.004160865089536750980, 0.004893036537146153858, 0.005625207984755555869, 0.006357379432364958748 ),
 .UNSPECIFIED. ) ;
#19008=DIRECTION ( 'NONE',  ( 1.000000000000000000, 0.000000000000000000, 1.613696256722611405E-16 ) ) ;
#19014=FACE_OUTER_BOUND ( 'NONE', #516, .T. ) ;
#19016=FACE_BOUND ( 'NONE', #13061, .T. ) ;
#19026=CARTESIAN_POINT ( 'NONE',  ( 27.94974746859769255, 27.94974746730969528, -29.00000000000000355 ) ) ;
#19044=VECTOR ( 'NONE', #16968, 1000.000000000000000 ) ;
#19062=CARTESIAN_POINT ( 'NONE',  ( 26.45000000029184051, 16.99999999900385461, -15.99999999999999289 ) ) ;
#19063=DIRECTION ( 'NONE',  ( -0.000000000000000000, 1.000000000000000000, 0.000000000000000000 ) ) ;
#19065=DIRECTION ( 'NONE',  ( -1.000000000000000000, 0.000000000000000000, 0.000000000000000000 ) ) ;
#19084=DIRECTION ( 'NONE',  ( -0.000000000000000000, -0.000000000000000000, 1.000000000000000000 ) ) ;
#19086=CARTESIAN_POINT ( 'NONE',  ( 6.000000000291855429, 2.999999999003851503, -8.549999999999998934 ) ) ;
#19100=DIRECTION ( 'NONE',  ( -0.000000000000000000, -0.000000000000000000, 1.000000000000000000 ) ) ;
#19112=CARTESIAN_POINT ( 'NONE',  ( 3.000000000291852764, 42.99999999900385461, -18.50000000000000355 ) ) ;
#19127=DIRECTION ( 'NONE',  ( 0.000000000000000000, -1.000000000000000000, 0.000000000000000000 ) ) ;
#19129=EDGE_LOOP ( 'NONE', ( #15308, #949, #4837, #3692 ) ) ;
#19136=VERTEX_POINT ( 'NONE', #18783 ) ;
#19146=EDGE_CURVE ( 'NONE', #84, #4283, #16994, .T. ) ;
#19147=CARTESIAN_POINT ( 'NONE',  ( -4.775149780314047909, 35.99999999900384751, -19.49999996803511237 ) ) ;
#19159=FACE_BOUND ( 'NONE', #17900, .T. ) ;
#19160=EDGE_CURVE ( 'NONE', #6752, #14012, #18936, .T. ) ;
#19174=ORIENTED_EDGE ( 'NONE', *, *, #12376, .F. ) ;
#19182=AXIS2_PLACEMENT_3D ( 'NONE', #11562, #11671, #8391 ) ;
#19191=VERTEX_POINT ( 'NONE', #18659 ) ;
#19202=EDGE_CURVE ( 'NONE', #22242, #343, #2544, .T. ) ;
#19222=B_SPLINE_CURVE_WITH_KNOTS ( 'NONE', 3,
 ( #13021, #561, #1370, #13720 ),
 .UNSPECIFIED., .F., .F.,
 ( 4, 4 ),
 ( 6.992893892674702526E-18, 1.060678621364840933E-05 ),
 .UNSPECIFIED. ) ;
#19223=VERTEX_POINT ( 'NONE', #7957 ) ;
#19232=DIRECTION ( 'NONE',  ( 1.000000000000000000, 0.000000000000000000, 0.000000000000000000 ) ) ;
#19241=PLANE ( 'NONE',  #674 ) ;
#19243=VERTEX_POINT ( 'NONE', #6555 ) ;
#19257=CARTESIAN_POINT ( 'NONE',  ( -5.523909222218111204, 35.99999999900384751, -19.02619312440723576 ) ) ;
#19261=AXIS2_PLACEMENT_3D ( 'NONE', #22537, #8300, #22417 ) ;
#19266=CARTESIAN_POINT ( 'NONE',  ( -6.999999999708156118, 6.999999999003851947, -15.99999999999999289 ) ) ;
#19272=EDGE_CURVE ( 'NONE', #11088, #10365, #20904, .T. ) ;
#19278=CARTESIAN_POINT ( 'NONE',  ( -5.311293330707327343, 35.99999999900384751, -25.93870558608502463 ) ) ;
#19288=ORIENTED_EDGE ( 'NONE', *, *, #21581, .F. ) ;
#19306=ORIENTED_EDGE ( 'NONE', *, *, #18726, .F. ) ;
#19310=EDGE_LOOP ( 'NONE', ( #21290, #689, #1915, #13362 ) ) ;
#19318=AXIS2_PLACEMENT_3D ( 'NONE', #22304, #13929, #21003 ) ;
#19321=DIRECTION ( 'NONE',  ( -0.000000000000000000, 1.000000000000000000, -0.000000000000000000 ) ) ;
#19322=CYLINDRICAL_SURFACE ( 'NONE', #7220, 6.999999999999999112 ) ;
#19336=DIRECTION ( 'NONE',  ( 0.000000000000000000, 0.000000000000000000, -1.000000000000000000 ) ) ;
#19341=EDGE_CURVE ( 'NONE', #5825, #19191, #7537, .T. ) ;
#19343=ORIENTED_EDGE ( 'NONE', *, *, #17273, .F. ) ;
#19354=DIRECTION ( 'NONE',  ( 0.000000000000000000, 0.000000000000000000, -1.000000000000000000 ) ) ;
#19360=CARTESIAN_POINT ( 'NONE',  ( -6.999999999708142795, 13.99999999900385106, -19.00000000000000355 ) ) ;
#19362=ORIENTED_EDGE ( 'NONE', *, *, #22942, .F. ) ;
#19371=VERTEX_POINT ( 'NONE', #22251 ) ;
#19375=LINE ( 'NONE', #6921, #22802 ) ;
#19376=CARTESIAN_POINT ( 'NONE',  ( -3.999999999708153453, 42.99999999900385461, -29.50000000000000000 ) ) ;
#19380=CARTESIAN_POINT ( 'NONE',  ( 30.00000000029184832, 2.999999999003851503, -45.00000000000000000 ) ) ;
#19390=ORIENTED_EDGE ( 'NONE', *, *, #21633, .F. ) ;
#19393=ORIENTED_EDGE ( 'NONE', *, *, #7816, .F. ) ;
#19413=( NAMED_UNIT ( * ) PLANE_ANGLE_UNIT ( ) SI_UNIT ( $, .RADIAN. ) );
#19414=EDGE_CURVE ( 'NONE', #14699, #9093, #18557, .T. ) ;
#19438=CIRCLE ( 'NONE', #17572, 1.000000000000000000 ) ;
#19442=EDGE_CURVE ( 'NONE', #22993, #14621, #16710, .T. ) ;
#19467=ORIENTED_EDGE ( 'NONE', *, *, #6670, .F. ) ;
#19472=CARTESIAN_POINT ( 'NONE',  ( 27.94974746859769255, 27.94974746730969528, -25.50000000000000355 ) ) ;
#19474=CARTESIAN_POINT ( 'NONE',  ( -6.960550854630938034, 36.00005224601466836, -26.48493219021591827 ) ) ;
#19477=CARTESIAN_POINT ( 'NONE',  ( 30.00000000029184832, 2.999999999003851503, -8.549999999999997158 ) ) ;
#19487=AXIS2_PLACEMENT_3D ( 'NONE', #12875, #14521, #2400 ) ;
#19498=VECTOR ( 'NONE', #5009, 1000.000000000000114 ) ;
#19510=ADVANCED_FACE ( 'NONE', ( #12141 ), #6282, .F. ) ;
#19517=CARTESIAN_POINT ( 'NONE',  ( -6.566827242015937038, 35.99999999936095207, -26.31323010872985435 ) ) ;
#19521=CARTESIAN_POINT ( 'NONE',  ( 35.50000000029185543, 16.99999999900385461, -19.00000000000000355 ) ) ;
#19531=DIRECTION ( 'NONE',  ( -1.000000000000000000, 0.000000000000000000, 0.000000000000000000 ) ) ;
#19562=DIRECTION ( 'NONE',  ( -0.000000000000000000, 1.000000000000000000, -0.000000000000000000 ) ) ;
#19572=VERTEX_POINT ( 'NONE', #18855 ) ;
#19611=EDGE_CURVE ( 'NONE', #19371, #17223, #9201, .T. ) ;
#19619=VECTOR ( 'NONE', #11855, 1000.000000000000000 ) ;
#19627=AXIS2_PLACEMENT_3D ( 'NONE', #14272, #21685, #16244 ) ;
#19643=LINE ( 'NONE', #6826, #13663 ) ;
#19646=PRODUCT_DEFINITION_SHAPE ( 'NONE', 'NONE',  #22880 ) ;
#19649=CYLINDRICAL_SURFACE ( 'NONE', #5922, 0.4999999999999982236 ) ;
#19669=DIRECTION ( 'NONE',  ( 0.000000000000000000, -1.000000000000000000, 0.000000000000000000 ) ) ;
#19677=VECTOR ( 'NONE', #2068, 1000.000000000000000 ) ;
#19696=VERTEX_POINT ( 'NONE', #7211 ) ;
#19704=ORIENTED_EDGE ( 'NONE', *, *, #16619, .F. ) ;
#19714=CARTESIAN_POINT ( 'NONE',  ( -6.959810536856680940, 36.00015702695179698, -26.48940942388196618 ) ) ;
#19716=VECTOR ( 'NONE', #9924, 1000.000000000000000 ) ;
#19730=ADVANCED_FACE ( 'NONE', ( #8736 ), #7681, .T. ) ;
#19738=ADVANCED_FACE ( 'NONE', ( #1683 ), #383, .F. ) ;
#19750=EDGE_CURVE ( 'NONE', #8991, #8999, #22130, .T. ) ;
#19786=CARTESIAN_POINT ( 'NONE',  ( -3.999999999708153453, 42.99999999900385461, -18.50000000000000355 ) ) ;
#19799=AXIS2_PLACEMENT_3D ( 'NONE', #739, #20505, #11427 ) ;
#19813=VERTEX_POINT ( 'NONE', #18957 ) ;
#19816=AXIS2_PLACEMENT_3D ( 'NONE', #11887, #4590, #22960 ) ;
#19822=DIRECTION ( 'NONE',  ( 0.000000000000000000, -1.000000000000000000, 0.000000000000000000 ) ) ;
#19828=VECTOR ( 'NONE', #15617, 1000.000000000000000 ) ;
#19843=CARTESIAN_POINT ( 'NONE',  ( 33.59619407800441593, 21.59619407671642222, -19.00000000000000355 ) ) ;
#19853=CARTESIAN_POINT ( 'NONE',  ( 3.000000000291852764, 42.99999999900385461, -25.50000000000000355 ) ) ;
#19881=CARTESIAN_POINT ( 'NONE',  ( 6.000000000291855429, 2.999999999003851503, -39.00000000000000000 ) ) ;
#19887=LINE ( 'NONE', #12347, #17981 ) ;
#19910=CARTESIAN_POINT ( 'NONE',  ( 2.918498775983380256E-10, 5.999999999003851059, -29.00000000000000355 ) ) ;
#19937=VERTEX_POINT ( 'NONE', #10231 ) ;
#19970=DIRECTION ( 'NONE',  ( 1.000000000000000000, 0.000000000000000000, 0.000000000000000000 ) ) ;
#19989=DIRECTION ( 'NONE',  ( 0.000000000000000000, 0.000000000000000000, -1.000000000000000000 ) ) ;
#19996=ADVANCED_FACE ( 'NONE', ( #7077 ), #23077, .F. ) ;
#20001=AXIS2_PLACEMENT_3D ( 'NONE', #22622, #10264, #8503 ) ;
#20016=LINE ( 'NONE', #3892, #7896 ) ;
#20043=VERTEX_POINT ( 'NONE', #17766 ) ;
#20044=ORIENTED_EDGE ( 'NONE', *, *, #16010, .F. ) ;
#20052=CYLINDRICAL_SURFACE ( 'NONE', #5444, 0.5000000000000004441 ) ;
#20061=DIRECTION ( 'NONE',  ( 0.000000000000000000, 0.000000000000000000, 1.000000000000000000 ) ) ;
#20065=CYLINDRICAL_SURFACE ( 'NONE', #18286, 3.000000000000000000 ) ;
#20073=ORIENTED_EDGE ( 'NONE', *, *, #22322, .F. ) ;
#20082=AXIS2_PLACEMENT_3D ( 'NONE', #22416, #14999, #13363 ) ;
#20094=DIRECTION ( 'NONE',  ( 0.000000000000000000, -1.000000000000000000, 0.000000000000000000 ) ) ;
#20099=CARTESIAN_POINT ( 'NONE',  ( -4.470458892752996682, 37.36863211987453326, -28.96516477595391592 ) ) ;
#20107=DIRECTION ( 'NONE',  ( -0.000000000000000000, -0.000000000000000000, 1.000000000000000000 ) ) ;
#20113=EDGE_LOOP ( 'NONE', ( #12710, #20073, #16942, #7509 ) ) ;
#20140=CARTESIAN_POINT ( 'NONE',  ( 2.918498775983380256E-10, 2.999999999003851503, -15.99999999999999289 ) ) ;
#20146=DIRECTION ( 'NONE',  ( -0.7071067811865475727, 0.7071067811865475727, 0.000000000000000000 ) ) ;
#20157=ORIENTED_EDGE ( 'NONE', *, *, #21508, .T. ) ;
#20174=CARTESIAN_POINT ( 'NONE',  ( 29.00000000029184832, 16.99999999900385461, -29.00000000000000355 ) ) ;
#20184=ORIENTED_EDGE ( 'NONE', *, *, #1058, .F. ) ;
#20194=ORIENTED_EDGE ( 'NONE', *, *, #4180, .T. ) ;
#20219=CARTESIAN_POINT ( 'NONE',  ( -4.149603749300068145, 38.03274690132711555, -28.99686245475831470 ) ) ;
#20240=CARTESIAN_POINT ( 'NONE',  ( 7.596194078004423034, 47.59619407671642222, -18.50000000000000355 ) ) ;
#20253=FACE_OUTER_BOUND ( 'NONE', #15312, .T. ) ;
#20260=CARTESIAN_POINT ( 'NONE',  ( 33.94974746859769255, 21.94974746730969528, -25.50000000000000355 ) ) ;
#20263=CARTESIAN_POINT ( 'NONE',  ( 2.918498775983380256E-10, 5.999999999003851059, -32.00000000000000000 ) ) ;
#20276=ORIENTED_EDGE ( 'NONE', *, *, #17482, .F. ) ;
#20279=VERTEX_POINT ( 'NONE', #11740 ) ;
#20298=CARTESIAN_POINT ( 'NONE',  ( 33.94974746859769255, 21.94974746730969528, -18.50000000000000355 ) ) ;
#20299=VECTOR ( 'NONE', #8041, 1000.000000000000000 ) ;
#20303=EDGE_CURVE ( 'NONE', #16865, #19136, #22698, .T. ) ;
#20313=LINE ( 'NONE', #4177, #21778 ) ;
#20314=VECTOR ( 'NONE', #2249, 1000.000000000000000 ) ;
#20329=ORIENTED_EDGE ( 'NONE', *, *, #5967, .F. ) ;
#20340=CARTESIAN_POINT ( 'NONE',  ( -6.959810536856695151, 36.00015702695179698, -18.51059057611807646 ) ) ;
#20375=DIRECTION ( 'NONE',  ( -0.000000000000000000, 1.000000000000000000, -0.000000000000000000 ) ) ;
#20377=ADVANCED_FACE ( 'NONE', ( #7046 ), #3281, .F. ) ;
#20379=ORIENTED_EDGE ( 'NONE', *, *, #21934, .F. ) ;
#20383=UNCERTAINTY_MEASURE_WITH_UNIT (LENGTH_MEASURE( 1.000000000000000082E-05 ), #17649, 'distance_accuracy_value', 'NONE');
#20397=VECTOR ( 'NONE', #19008, 1000.000000000000000 ) ;
#20426=ORIENTED_EDGE ( 'NONE', *, *, #3231, .T. ) ;
#20454=EDGE_CURVE ( 'NONE', #19937, #4283, #15733, .T. ) ;
#20456=ORIENTED_EDGE ( 'NONE', *, *, #4682, .T. ) ;
#20460=EDGE_CURVE ( 'NONE', #19191, #16629, #1845, .T. ) ;
#20464=CARTESIAN_POINT ( 'NONE',  ( 6.000000000291855429, 2.999999999003851503, -5.999999999999998224 ) ) ;
#20487=DIRECTION ( 'NONE',  ( 1.000000000000000000, 0.000000000000000000, 0.000000000000000000 ) ) ;
#20488=ORIENTED_EDGE ( 'NONE', *, *, #6241, .T. ) ;
#20491=CARTESIAN_POINT ( 'NONE',  ( 6.000000000291855429, -0.5000000009961480529, -39.00000000000000000 ) ) ;
#20493=CARTESIAN_POINT ( 'NONE',  ( -4.149603749300068145, 38.03274690132714397, -16.00313754524167109 ) ) ;
#20505=DIRECTION ( 'NONE',  ( -0.000000000000000000, 1.000000000000000000, -0.000000000000000000 ) ) ;
#20511=ORIENTED_EDGE ( 'NONE', *, *, #14303, .T. ) ;
#20516=CARTESIAN_POINT ( 'NONE',  ( 36.00000000029184832, 2.999999999003851503, -12.99999999999999822 ) ) ;
#20520=LINE ( 'NONE', #14976, #889 ) ;
#20521=LINE ( 'NONE', #15322, #20299 ) ;
#20531=CARTESIAN_POINT ( 'NONE',  ( -5.454524251050743899, 13.82936183575430356, -28.63121289012828186 ) ) ;
#20535=ORIENTED_EDGE ( 'NONE', *, *, #11533, .F. ) ;
#20540=ORIENTED_EDGE ( 'NONE', *, *, #3494, .T. ) ;
#20544=FACE_OUTER_BOUND ( 'NONE', #21807, .T. ) ;
#20546=DIRECTION ( 'NONE',  ( -0.000000000000000000, -1.000000000000000000, 0.000000000000000000 ) ) ;
#20559=ORIENTED_EDGE ( 'NONE', *, *, #21633, .T. ) ;
#20565=PRODUCT ( 'Base', 'Base', '', ( #2236 ) ) ;
#20572=AXIS2_PLACEMENT_3D ( 'NONE', #11842, #11714, #10306 ) ;
#20590=CIRCLE ( 'NONE', #6682, 0.4999999999999982236 ) ;
#20633=CARTESIAN_POINT ( 'NONE',  ( -3.999999999708153453, 13.99999999900385106, -19.50000000000000355 ) ) ;
#20641=CYLINDRICAL_SURFACE ( 'NONE', #16612, 2.999999999999999112 ) ;
#20648=CARTESIAN_POINT ( 'NONE',  ( -6.230270079314315090, 13.95903802731504584, -28.01626849522005358 ) ) ;
#20662=EDGE_CURVE ( 'NONE', #5983, #1520, #18081, .T. ) ;
#20670=DIRECTION ( 'NONE',  ( 0.000000000000000000, -0.000000000000000000, -1.000000000000000000 ) ) ;
#20682=FACE_BOUND ( 'NONE', #17870, .T. ) ;
#20695=CARTESIAN_POINT ( 'NONE',  ( 7.596194078004423034, 47.59619407671642222, -26.50000000000000000 ) ) ;
#20700=DIRECTION ( 'NONE',  ( -0.000000000000000000, -1.000000000000000000, 0.000000000000000000 ) ) ;
#20703=PLANE ( 'NONE',  #16370 ) ;
#20708=ORIENTED_EDGE ( 'NONE', *, *, #5574, .T. ) ;
#20709=ORIENTED_EDGE ( 'NONE', *, *, #22981, .F. ) ;
#20720=DIRECTION ( 'NONE',  ( 0.000000000000000000, 0.000000000000000000, 1.000000000000000000 ) ) ;
#20760=CYLINDRICAL_SURFACE ( 'NONE', #16600, 0.5000000000000004441 ) ;
#20778=AXIS2_PLACEMENT_3D ( 'NONE', #20898, #2888, #6427 ) ;
#20781=ORIENTED_EDGE ( 'NONE', *, *, #2773, .F. ) ;
#20796=AXIS2_PLACEMENT_3D ( 'NONE', #5091, #21679, #8973 ) ;
#20797=DIRECTION ( 'NONE',  ( 0.000000000000000000, 0.000000000000000000, -1.000000000000000000 ) ) ;
#20798=VECTOR ( 'NONE', #15110, 1000.000000000000000 ) ;
#20802=VECTOR ( 'NONE', #6394, 1000.000000000000000 ) ;
#20817=AXIS2_PLACEMENT_3D ( 'NONE', #1500, #21271, #3611 ) ;
#20834=CARTESIAN_POINT ( 'NONE',  ( 2.918498775983380256E-10, 2.999999999003851503, -26.00000000000000000 ) ) ;
#20841=DIRECTION ( 'NONE',  ( 1.613696256722611405E-16, -0.000000000000000000, 1.000000000000000000 ) ) ;
#20843=DIRECTION ( 'NONE',  ( 0.000000000000000000, 0.000000000000000000, -1.000000000000000000 ) ) ;
#20844=AXIS2_PLACEMENT_3D ( 'NONE', #13571, #8619, #11673 ) ;
#20848=CARTESIAN_POINT ( 'NONE',  ( -3.999999999708153453, 13.99999999900385106, -19.50000000000000355 ) ) ;
#20849=AXIS2_PLACEMENT_3D ( 'NONE', #3243, #8642, #15686 ) ;
#20863=ORIENTED_EDGE ( 'NONE', *, *, #20987, .T. ) ;
#20877=DIRECTION ( 'NONE',  ( 1.000000000000000000, 0.000000000000000000, 0.000000000000000000 ) ) ;
#20882=EDGE_CURVE ( 'NONE', #13641, #4111, #3283, .T. ) ;
#20898=CARTESIAN_POINT ( 'NONE',  ( 3.000000000291852764, 42.99999999900385461, -29.00000000000000355 ) ) ;
#20903=FACE_OUTER_BOUND ( 'NONE', #4282, .T. ) ;
#20904=LINE ( 'NONE', #6898, #17421 ) ;
#20909=EDGE_CURVE ( 'NONE', #4111, #13641, #22066, .T. ) ;
#20912=DIRECTION ( 'NONE',  ( 0.000000000000000000, -0.000000000000000000, -1.000000000000000000 ) ) ;
#20913=VERTEX_POINT ( 'NONE', #17409 ) ;
#20933=CARTESIAN_POINT ( 'NONE',  ( 30.00000000029184832, -0.5000000009961480529, -3.449999999999999289 ) ) ;
#20935=DIRECTION ( 'NONE',  ( 1.000000000000000000, 0.000000000000000000, 0.000000000000000000 ) ) ;
#20941=CIRCLE ( 'NONE', #21318, 0.5000000000000004441 ) ;
#20943=ORIENTED_EDGE ( 'NONE', *, *, #2887, .T. ) ;
#20947=CARTESIAN_POINT ( 'NONE',  ( -4.751720029897110287, 36.43339712399804853, -26.00000000000000711 ) ) ;
#20948=AXIS2_PLACEMENT_3D ( 'NONE', #19266, #1061, #3169 ) ;
#20951=DIRECTION ( 'NONE',  ( 1.000000000000000000, 0.000000000000000000, 0.000000000000000000 ) ) ;
#20965=AXIS2_PLACEMENT_3D ( 'NONE', #22633, #13700, #20877 ) ;
#20987=EDGE_CURVE ( 'NONE', #7942, #15111, #10134, .T. ) ;
#20993=( GEOMETRIC_REPRESENTATION_CONTEXT ( 3 ) GLOBAL_UNCERTAINTY_ASSIGNED_CONTEXT ( ( #20383 ) ) GLOBAL_UNIT_ASSIGNED_CONTEXT ( ( #17649, #22724, #23087 ) ) REPRESENTATION_CONTEXT ( 'NONE', 'WORKASPACE' ) );
#20997=EDGE_LOOP ( 'NONE', ( #18156, #827 ) ) ;
#20999=CIRCLE ( 'NONE', #10844, 2.550000000000002043 ) ;
#21003=DIRECTION ( 'NONE',  ( 1.000000000000000000, 0.000000000000000000, 0.000000000000000000 ) ) ;
#21021=EDGE_CURVE ( 'NONE', #17223, #555, #15532, .T. ) ;
#21041=CARTESIAN_POINT ( 'NONE',  ( -6.525563119752677999, 36.00216957434000165, -18.62502167978186307 ) ) ;
#21054=EDGE_CURVE ( 'NONE', #20043, #13206, #20941, .T. ) ;
#21058=CARTESIAN_POINT ( 'NONE',  ( -4.550510256924974684, 35.99999999900384751, -25.50000000000000000 ) ) ;
#21064=DIRECTION ( 'NONE',  ( 0.000000000000000000, 0.000000000000000000, 1.000000000000000000 ) ) ;
#21069=CARTESIAN_POINT ( 'NONE',  ( -6.999999999708142795, 13.99999999900385106, -22.50000000000000000 ) ) ;
#21086=AXIS2_PLACEMENT_3D ( 'NONE', #14214, #12432, #17857 ) ;
#21093=CARTESIAN_POINT ( 'NONE',  ( 29.00000000029184832, 16.99999999900385461, -19.49999999999998934 ) ) ;
#21095=CARTESIAN_POINT ( 'NONE',  ( 6.000000000291855429, 2.999999999003851503, -36.44999999999999574 ) ) ;
#21101=EDGE_CURVE ( 'NONE', #4567, #14963, #7532, .T. ) ;
#21161=AXIS2_PLACEMENT_3D ( 'NONE', #11224, #16615, #15438 ) ;
#21167=DIRECTION ( 'NONE',  ( 0.000000000000000000, 1.000000000000000000, 0.000000000000000000 ) ) ;
#21170=EDGE_LOOP ( 'NONE', ( #22730, #8826, #1413, #8820 ) ) ;
#21178=CARTESIAN_POINT ( 'NONE',  ( -4.904729001339799943, 35.99999999900385461, -25.92290237457175905 ) ) ;
#21200=AXIS2_PLACEMENT_3D ( 'NONE', #21839, #5617, #13133 ) ;
#21209=ORIENTED_EDGE ( 'NONE', *, *, #2930, .F. ) ;
#21211=VECTOR ( 'NONE', #18610, 1000.000000000000000 ) ;
#21215=CIRCLE ( 'NONE', #16661, 2.550000000000003819 ) ;
#21218=CIRCLE ( 'NONE', #19318, 2.550000000000002043 ) ;
#21220=LINE ( 'NONE', #3438, #21938 ) ;
#21222=EDGE_CURVE ( 'NONE', #555, #14256, #13523, .T. ) ;
#21234=DIRECTION ( 'NONE',  ( 0.000000000000000000, 0.000000000000000000, -1.000000000000000000 ) ) ;
#21236=VERTEX_POINT ( 'NONE', #12078 ) ;
#21243=ADVANCED_FACE ( 'NONE', ( #6694, #19159, #10210 ), #20703, .F. ) ;
#21246=VECTOR ( 'NONE', #13751, 1000.000000000000000 ) ;
#21247=CARTESIAN_POINT ( 'NONE',  ( 36.00000000029184832, 5.999999999003851059, -16.00000000000000000 ) ) ;
#21271=DIRECTION ( 'NONE',  ( 0.000000000000000000, 0.000000000000000000, -1.000000000000000000 ) ) ;
#21277=FACE_OUTER_BOUND ( 'NONE', #13759, .T. ) ;
#21290=ORIENTED_EDGE ( 'NONE', *, *, #2313, .T. ) ;
#21306=CARTESIAN_POINT ( 'NONE',  ( -6.999999999708142795, 49.99999999900385461, -26.00000000000000711 ) ) ;
#21314=AXIS2_PLACEMENT_3D ( 'NONE', #8215, #10095, #12065 ) ;
#21318=AXIS2_PLACEMENT_3D ( 'NONE', #9060, #10708, #5541 ) ;
#21324=ORIENTED_EDGE ( 'NONE', *, *, #18037, .F. ) ;
#21328=CARTESIAN_POINT ( 'NONE',  ( -5.623500955413153868, 35.99999999900385461, -25.73132293306449370 ) ) ;
#21333=AXIS2_PLACEMENT_3D ( 'NONE', #2685, #2229, #4102 ) ;
#21338=EDGE_CURVE ( 'NONE', #18076, #4111, #6806, .T. ) ;
#21353=EDGE_CURVE ( 'NONE', #1834, #4926, #5880, .T. ) ;
#21365=DIRECTION ( 'NONE',  ( 1.000000000000000000, 0.000000000000000000, 0.000000000000000000 ) ) ;
#21369=ORIENTED_EDGE ( 'NONE', *, *, #1628, .T. ) ;
#21372=DIRECTION ( 'NONE',  ( -1.000000000000000000, 0.000000000000000000, 0.000000000000000000 ) ) ;
#21375=CARTESIAN_POINT ( 'NONE',  ( 36.00000000029184832, 16.99999999900385461, -18.50000000000000355 ) ) ;
#21381=CARTESIAN_POINT ( 'NONE',  ( 29.00000000029184832, 16.99999999900385461, -29.00000000000000355 ) ) ;
#21392=ORIENTED_EDGE ( 'NONE', *, *, #20303, .F. ) ;
#21394=CARTESIAN_POINT ( 'NONE',  ( -3.999999999708139686, 49.99999999900386172, -29.00000000000000355 ) ) ;
#21405=DIRECTION ( 'NONE',  ( 0.000000000000000000, 0.000000000000000000, 1.000000000000000000 ) ) ;
#21417=CARTESIAN_POINT ( 'NONE',  ( -4.993857080232831258, 35.99999999900384751, -25.53590495946178152 ) ) ;
#21448=CYLINDRICAL_SURFACE ( 'NONE', #5836, 2.999999999999999112 ) ;
#21449=EDGE_CURVE ( 'NONE', #15111, #688, #2431, .T. ) ;
#21463=DIRECTION ( 'NONE',  ( 0.000000000000000000, 0.000000000000000000, 1.000000000000000000 ) ) ;
#21468=ORIENTED_EDGE ( 'NONE', *, *, #10960, .T. ) ;
#21469=EDGE_LOOP ( 'NONE', ( #17453, #15449, #10145, #20456 ) ) ;
#21476=EDGE_CURVE ( 'NONE', #14170, #12207, #18647, .T. ) ;
#21484=DIRECTION ( 'NONE',  ( -0.000000000000000000, -0.000000000000000000, -1.000000000000000000 ) ) ;
#21508=EDGE_CURVE ( 'NONE', #7853, #8658, #7958, .T. ) ;
#21509=DIRECTION ( 'NONE',  ( 1.000000000000000000, 0.000000000000000000, -1.613696256722611405E-16 ) ) ;
#21511=CIRCLE ( 'NONE', #19627, 2.550000000000003819 ) ;
#21548=AXIS2_PLACEMENT_3D ( 'NONE', #2839, #9899, #17405 ) ;
#21581=EDGE_CURVE ( 'NONE', #22262, #3520, #16887, .T. ) ;
#21593=ORIENTED_EDGE ( 'NONE', *, *, #9415, .F. ) ;
#21598=CARTESIAN_POINT ( 'NONE',  ( 2.918498775983380256E-10, 5.999999999003851059, -12.99999999999999822 ) ) ;
#21615=AXIS2_PLACEMENT_3D ( 'NONE', #16120, #22856, #3559 ) ;
#21633=EDGE_CURVE ( 'NONE', #19696, #8999, #14154, .T. ) ;
#21634=LINE ( 'NONE', #7386, #15313 ) ;
#21637=CARTESIAN_POINT ( 'NONE',  ( 36.00000000029184832, 16.99999999900385461, -25.50000000000000355 ) ) ;
#21641=ORIENTED_EDGE ( 'NONE', *, *, #17447, .T. ) ;
#21656=CARTESIAN_POINT ( 'NONE',  ( -6.961281259571826752, 35.99999999900384751, -18.51954822859009653 ) ) ;
#21657=VECTOR ( 'NONE', #9525, 1000.000000000000000 ) ;
#21658=CARTESIAN_POINT ( 'NONE',  ( -6.999999999708142795, 36.49999999900384751, -19.50000000000000355 ) ) ;
#21659=DIRECTION ( 'NONE',  ( 0.7071067811865475727, -0.7071067811865475727, 0.000000000000000000 ) ) ;
#21666=EDGE_CURVE ( 'NONE', #14655, #2319, #14071, .T. ) ;
#21667=ORIENTED_EDGE ( 'NONE', *, *, #9405, .T. ) ;
#21669=ADVANCED_FACE ( 'NONE', ( #23260 ), #10536, .F. ) ;
#21674=DIRECTION ( 'NONE',  ( 0.000000000000000000, 0.000000000000000000, -1.000000000000000000 ) ) ;
#21679=DIRECTION ( 'NONE',  ( 0.000000000000000000, -1.000000000000000000, 0.000000000000000000 ) ) ;
#21682=AXIS2_PLACEMENT_3D ( 'NONE', #6574, #1163, #13853 ) ;
#21685=DIRECTION ( 'NONE',  ( -0.000000000000000000, -1.000000000000000000, -0.000000000000000000 ) ) ;
#21698=VECTOR ( 'NONE', #13967, 1000.000000000000000 ) ;
#21707=DIRECTION ( 'NONE',  ( 0.000000000000000000, 0.000000000000000000, -1.000000000000000000 ) ) ;
#21716=VECTOR ( 'NONE', #944, 1000.000000000000000 ) ;
#21733=ADVANCED_FACE ( 'NONE', ( #2054 ), #20065, .F. ) ;
#21754=DIRECTION ( 'NONE',  ( 0.000000000000000000, 0.000000000000000000, 1.000000000000000000 ) ) ;
#21767=CARTESIAN_POINT ( 'NONE',  ( 29.00000000029184832, 16.99999999900385461, -15.99999999999999289 ) ) ;
#21768=CARTESIAN_POINT ( 'NONE',  ( -6.962001439796694058, 35.99999999900384751, -18.52402997057235723 ) ) ;
#21771=EDGE_CURVE ( 'NONE', #888, #3083, #7588, .T. ) ;
#21778=VECTOR ( 'NONE', #7494, 1000.000000000000000 ) ;
#21781=ORIENTED_EDGE ( 'NONE', *, *, #12553, .T. ) ;
#21783=PRODUCT_DEFINITION_FORMATION_WITH_SPECIFIED_SOURCE ( 'ANY', '', #20565, .NOT_KNOWN. ) ;
#21795=CARTESIAN_POINT ( 'NONE',  ( -6.958039891257955745, 36.00029345514013102, -18.49999999999999645 ) ) ;
#21801=LINE ( 'NONE', #12489, #9483 ) ;
#21807=EDGE_LOOP ( 'NONE', ( #16516, #7477, #9305, #21209 ) ) ;
#21809=ORIENTED_EDGE ( 'NONE', *, *, #8180, .F. ) ;
#21821=EDGE_CURVE ( 'NONE', #12647, #19572, #194, .T. ) ;
#21829=CARTESIAN_POINT ( 'NONE',  ( 7.949747468597695210, 47.94974746730969173, -25.50000000000000355 ) ) ;
#21832=ORIENTED_EDGE ( 'NONE', *, *, #4981, .T. ) ;
#21839=CARTESIAN_POINT ( 'NONE',  ( 30.00000000029184832, 2.999999999003851503, -5.999999999999998224 ) ) ;
#21856=AXIS2_PLACEMENT_3D ( 'NONE', #14065, #3253, #4998 ) ;
#21859=ORIENTED_EDGE ( 'NONE', *, *, #22185, .F. ) ;
#21860=CARTESIAN_POINT ( 'NONE',  ( -6.525612274168519633, 36.03379296756838812, -27.63750043262194112 ) ) ;
#21865=LINE ( 'NONE', #22217, #22648 ) ;
#21901=CARTESIAN_POINT ( 'NONE',  ( -3.999999999708153453, 38.99999999900385461, -15.99999999999999289 ) ) ;
#21917=LINE ( 'NONE', #18044, #16795 ) ;
#21926=ORIENTED_EDGE ( 'NONE', *, *, #9090, .F. ) ;
#21931=VECTOR ( 'NONE', #18230, 1000.000000000000000 ) ;
#21934=EDGE_CURVE ( 'NONE', #15365, #7853, #2132, .T. ) ;
#21938=VECTOR ( 'NONE', #8612, 1000.000000000000000 ) ;
#21943=FACE_OUTER_BOUND ( 'NONE', #14404, .T. ) ;
#21945=CARTESIAN_POINT ( 'NONE',  ( -6.999999999708142795, 13.99999999900385106, -26.00000000000000000 ) ) ;
#21947=CARTESIAN_POINT ( 'NONE',  ( 30.00000000029184832, 2.999999999003851503, -36.45000000000000284 ) ) ;
#21953=CARTESIAN_POINT ( 'NONE',  ( 36.00000000029184832, 5.999999999003851059, -32.00000000000000000 ) ) ;
#21966=DIRECTION ( 'NONE',  ( 0.000000000000000000, 0.000000000000000000, -1.000000000000000000 ) ) ;
#21968=CARTESIAN_POINT ( 'NONE',  ( 2.918498775983380256E-10, 2.999999999003851503, -45.00000000000000000 ) ) ;
#21984=CARTESIAN_POINT ( 'NONE',  ( -5.549486778972979373, 36.19267127072042456, -18.86553880985036358 ) ) ;
#22000=FACE_OUTER_BOUND ( 'NONE', #17595, .T. ) ;
#22017=DIRECTION ( 'NONE',  ( -0.000000000000000000, 1.000000000000000000, 0.000000000000000000 ) ) ;
#22024=ORIENTED_EDGE ( 'NONE', *, *, #17482, .T. ) ;
#22031=ORIENTED_EDGE ( 'NONE', *, *, #17331, .T. ) ;
#22035=CYLINDRICAL_SURFACE ( 'NONE', #11739, 2.550000000000003819 ) ;
#22051=DIRECTION ( 'NONE',  ( 0.000000000000000000, -1.000000000000000000, 0.000000000000000000 ) ) ;
#22066=CIRCLE ( 'NONE', #19816, 2.549999999999996714 ) ;
#22094=CARTESIAN_POINT ( 'NONE',  ( 36.00000000029184832, -9.961476088449217059E-10, -18.50000000000000355 ) ) ;
#22115=AXIS2_PLACEMENT_3D ( 'NONE', #4943, #2963, #5306 ) ;
#22130=LINE ( 'NONE', #20260, #12166 ) ;
#22137=VECTOR ( 'NONE', #11759, 1000.000000000000000 ) ;
#22142=EDGE_CURVE ( 'NONE', #1547, #11088, #9281, .T. ) ;
#22152=ORIENTED_EDGE ( 'NONE', *, *, #16395, .T. ) ;
#22153=DIRECTION ( 'NONE',  ( 0.000000000000000000, 1.000000000000000000, 0.000000000000000000 ) ) ;
#22157=CARTESIAN_POINT ( 'NONE',  ( -4.499999999708154341, 35.49999999900384751, -22.50000000000000000 ) ) ;
#22161=CARTESIAN_POINT ( 'NONE',  ( 6.000000000291855429, 2.999999999003851503, -41.55000000000000426 ) ) ;
#22185=EDGE_CURVE ( 'NONE', #11088, #1547, #4378, .T. ) ;
#22193=CARTESIAN_POINT ( 'NONE',  ( 6.000000000291855429, -9.961476088449217059E-10, -45.00000000000000000 ) ) ;
#22195=CARTESIAN_POINT ( 'NONE',  ( -3.499999999708153453, 35.49999999900384751, -25.50000000000000000 ) ) ;
#22202=EDGE_CURVE ( 'NONE', #7853, #9785, #9646, .T. ) ;
#22217=CARTESIAN_POINT ( 'NONE',  ( -3.999999999708153453, 35.99999999900384751, -18.50000000000000355 ) ) ;
#22237=CIRCLE ( 'NONE', #12059, 0.5000000000000004441 ) ;
#22242=VERTEX_POINT ( 'NONE', #7787 ) ;
#22243=CARTESIAN_POINT ( 'NONE',  ( 7.949747468597695210, 47.94974746730969173, -19.49999999999998934 ) ) ;
#22246=CARTESIAN_POINT ( 'NONE',  ( -6.056833031243687770, 36.14537244600960975, -16.80371197567150432 ) ) ;
#22251=CARTESIAN_POINT ( 'NONE',  ( -4.550510256924974684, 35.99999999900384751, -19.50000000000000355 ) ) ;
#22260=ORIENTED_EDGE ( 'NONE', *, *, #2623, .F. ) ;
#22262=VERTEX_POINT ( 'NONE', #16825 ) ;
#22268=DIRECTION ( 'NONE',  ( 0.000000000000000000, 0.000000000000000000, 1.000000000000000000 ) ) ;
#22269=VERTEX_POINT ( 'NONE', #12440 ) ;
#22277=CARTESIAN_POINT ( 'NONE',  ( -6.999999999708142795, 35.99999999900384751, -19.00000000000000355 ) ) ;
#22304=CARTESIAN_POINT ( 'NONE',  ( 3.000000000291852764, 42.99999999900385461, -15.99999999999999289 ) ) ;
#22311=CIRCLE ( 'NONE', #4253, 5.999999999999998224 ) ;
#22322=EDGE_CURVE ( 'NONE', #14012, #12387, #17869, .T. ) ;
#22343=CARTESIAN_POINT ( 'NONE',  ( -5.631870895240913555, 35.99999999900384751, -19.26529513898303847 ) ) ;
#22350=VECTOR ( 'NONE', #4497, 1000.000000000000000 ) ;
#22351=DIRECTION ( 'NONE',  ( 0.000000000000000000, 0.000000000000000000, -1.000000000000000000 ) ) ;
#22354=DIRECTION ( 'NONE',  ( 0.000000000000000000, 0.000000000000000000, 1.000000000000000000 ) ) ;
#22364=CYLINDRICAL_SURFACE ( 'NONE', #2760, 3.000000000000000000 ) ;
#22367=ORIENTED_EDGE ( 'NONE', *, *, #19146, .F. ) ;
#22373=DIRECTION ( 'NONE',  ( 0.000000000000000000, 0.000000000000000000, -1.000000000000000000 ) ) ;
#22384=VERTEX_POINT ( 'NONE', #7733 ) ;
#22386=EDGE_LOOP ( 'NONE', ( #1802, #22367, #16198, #19288 ) ) ;
#22387=EDGE_LOOP ( 'NONE', ( #13761, #16746, #10659, #10862 ) ) ;
#22402=CARTESIAN_POINT ( 'NONE',  ( 7.949747468597695210, 47.94974746730969173, -26.50000000000000000 ) ) ;
#22409=ORIENTED_EDGE ( 'NONE', *, *, #19272, .T. ) ;
#22416=CARTESIAN_POINT ( 'NONE',  ( 6.000000000291855429, -9.961476088449217059E-10, -5.999999999999998224 ) ) ;
#22417=DIRECTION ( 'NONE',  ( 0.000000000000000000, 0.000000000000000000, -1.000000000000000000 ) ) ;
#22418=EDGE_LOOP ( 'NONE', ( #19306, #19362 ) ) ;
#22422=DIRECTION ( 'NONE',  ( 0.000000000000000000, -1.000000000000000000, 0.000000000000000000 ) ) ;
#22431=VERTEX_POINT ( 'NONE', #2550 ) ;
#22435=CIRCLE ( 'NONE', #12273, 0.5000000000000004441 ) ;
#22439=ORIENTED_EDGE ( 'NONE', *, *, #8097, .T. ) ;
#22444=ORIENTED_EDGE ( 'NONE', *, *, #16903, .T. ) ;
#22474=VERTEX_POINT ( 'NONE', #18437 ) ;
#22507=ADVANCED_FACE ( 'NONE', ( #20682, #15131, #15477 ), #19241, .F. ) ;
#22513=FACE_OUTER_BOUND ( 'NONE', #4358, .T. ) ;
#22537=CARTESIAN_POINT ( 'NONE',  ( 30.00000000029184832, -0.5000000009961480529, -39.00000000000000000 ) ) ;
#22557=VERTEX_POINT ( 'NONE', #15364 ) ;
#22559=ORIENTED_EDGE ( 'NONE', *, *, #4345, .T. ) ;
#22562=ORIENTED_EDGE ( 'NONE', *, *, #4336, .T. ) ;
#22567=CARTESIAN_POINT ( 'NONE',  ( -4.896882909245229953, 36.38534960922553552, -18.98204752465805356 ) ) ;
#22576=EDGE_CURVE ( 'NONE', #19223, #8999, #8203, .T. ) ;
#22587=DIRECTION ( 'NONE',  ( 1.000000000000000000, 0.000000000000000000, 0.000000000000000000 ) ) ;
#22589=AXIS2_PLACEMENT_3D ( 'NONE', #21767, #16447, #12458 ) ;
#22595=ADVANCED_FACE ( 'NONE', ( #1034 ), #11949, .F. ) ;
#22608=ADVANCED_FACE ( 'NONE', ( #12054 ), #16050, .T. ) ;
#22615=ORIENTED_EDGE ( 'NONE', *, *, #10614, .T. ) ;
#22618=( NAMED_UNIT ( * ) PLANE_ANGLE_UNIT ( ) SI_UNIT ( $, .RADIAN. ) );
#22622=CARTESIAN_POINT ( 'NONE',  ( 30.00000000029184832, 2.999999999003851503, -39.00000000000000000 ) ) ;
#22633=CARTESIAN_POINT ( 'NONE',  ( 3.000000000291852764, 42.99999999900385461, -45.00000000000000000 ) ) ;
#22634=CARTESIAN_POINT ( 'NONE',  ( -6.359599319592073030, 13.97158350606811617, -27.86358591318706246 ) ) ;
#22646=CIRCLE ( 'NONE', #10238, 0.5000000000000004441 ) ;
#22648=VECTOR ( 'NONE', #13508, 1000.000000000000000 ) ;
#22672=EDGE_LOOP ( 'NONE', ( #13812, #9854, #17094, #1857 ) ) ;
#22691=CARTESIAN_POINT ( 'NONE',  ( -6.999999999708142795, 38.99999999900385461, -26.50000000000000000 ) ) ;
#22698=LINE ( 'NONE', #819, #21246 ) ;
#22699=LINE ( 'NONE', #1169, #21698 ) ;
#22707=ORIENTED_EDGE ( 'NONE', *, *, #7654, .T. ) ;
#22710=CARTESIAN_POINT ( 'NONE',  ( -4.499999999708154341, 35.99999999900384751, -25.50000000000000000 ) ) ;
#22719=CARTESIAN_POINT ( 'NONE',  ( 26.09619407800442659, 29.09619407671642222, -19.00000000000000355 ) ) ;
#22724=( NAMED_UNIT ( * ) PLANE_ANGLE_UNIT ( ) SI_UNIT ( $, .RADIAN. ) );
#22730=ORIENTED_EDGE ( 'NONE', *, *, #18726, .T. ) ;
#22751=DIRECTION ( 'NONE',  ( 0.000000000000000000, 0.000000000000000000, 1.000000000000000000 ) ) ;
#22752=EDGE_CURVE ( 'NONE', #2725, #14653, #15924, .T. ) ;
#22761=VERTEX_POINT ( 'NONE', #2749 ) ;
#22778=FACE_BOUND ( 'NONE', #775, .T. ) ;
#22802=VECTOR ( 'NONE', #21509, 1000.000000000000000 ) ;
#22851=ORIENTED_EDGE ( 'NONE', *, *, #20909, .T. ) ;
#22856=DIRECTION ( 'NONE',  ( -1.000000000000000000, 0.000000000000000000, 1.734723475976805319E-15 ) ) ;
#22857=CARTESIAN_POINT ( 'NONE',  ( 36.00000000029184832, -9.961476088449217059E-10, -39.00000000000000000 ) ) ;
#22869=DIRECTION ( 'NONE',  ( 0.000000000000000000, -1.000000000000000000, 0.000000000000000000 ) ) ;
#22880=PRODUCT_DEFINITION ( 'UNKNOWN', '', #21783, #4161 ) ;
#22886=ADVANCED_FACE ( 'NONE', ( #6996 ), #11188, .F. ) ;
#22894=CARTESIAN_POINT ( 'NONE',  ( -6.959227345695446765, 36.00023956896081501, -26.49293639998818506 ) ) ;
#22938=EDGE_CURVE ( 'NONE', #9093, #14699, #13074, .T. ) ;
#22941=EDGE_LOOP ( 'NONE', ( #2149, #7538, #17102, #6189 ) ) ;
#22942=EDGE_CURVE ( 'NONE', #4090, #12296, #2938, .T. ) ;
#22946=ORIENTED_EDGE ( 'NONE', *, *, #3386, .F. ) ;
#22947=ORIENTED_EDGE ( 'NONE', *, *, #12246, .F. ) ;
#22949=ORIENTED_EDGE ( 'NONE', *, *, #13980, .F. ) ;
#22953=ORIENTED_EDGE ( 'NONE', *, *, #8180, .T. ) ;
#22956=PLANE ( 'NONE',  #10178 ) ;
#22960=DIRECTION ( 'NONE',  ( 0.000000000000000000, 0.000000000000000000, -1.000000000000000000 ) ) ;
#22961=SURFACE_STYLE_FILL_AREA ( #12113 ) ;
#22970=EDGE_LOOP ( 'NONE', ( #13231, #8632 ) ) ;
#22971=CIRCLE ( 'NONE', #13219, 3.499999999999999556 ) ;
#22975=CARTESIAN_POINT ( 'NONE',  ( -6.999999999708156118, 6.999999999003851947, -26.00000000000000000 ) ) ;
#22976=FACE_OUTER_BOUND ( 'NONE', #16029, .T. ) ;
#22981=EDGE_CURVE ( 'NONE', #14201, #19371, #5576, .T. ) ;
#22984=CARTESIAN_POINT ( 'NONE',  ( 3.000000000291852764, 42.99999999900385461, -29.00000000000000355 ) ) ;
#22990=CARTESIAN_POINT ( 'NONE',  ( 29.00000000029184832, 16.99999999900385461, -18.50000000000000355 ) ) ;
#22993=VERTEX_POINT ( 'NONE', #3789 ) ;
#23020=ORIENTED_EDGE ( 'NONE', *, *, #4648, .F. ) ;
#23024=CIRCLE ( 'NONE', #7240, 2.549999999999998934 ) ;
#23037=ADVANCED_FACE ( 'NONE', ( #7449 ), #7560, .F. ) ;
#23059=EDGE_CURVE ( 'NONE', #3643, #84, #21917, .T. ) ;
#23061=CARTESIAN_POINT ( 'NONE',  ( -5.471017171483509856, 36.21317998574328811, -26.11735242742819452 ) ) ;
#23064=EDGE_CURVE ( 'NONE', #22431, #8991, #20590, .T. ) ;
#23077=CYLINDRICAL_SURFACE ( 'NONE', #5457, 0.5000000000000004441 ) ;
#23081=VECTOR ( 'NONE', #14752, 1000.000000000000000 ) ;
#23085=DIRECTION ( 'NONE',  ( -0.000000000000000000, -0.000000000000000000, -1.000000000000000000 ) ) ;
#23087=( NAMED_UNIT ( * ) SI_UNIT ( $, .STERADIAN. ) SOLID_ANGLE_UNIT ( ) );
#23096=AXIS2_PLACEMENT_3D ( 'NONE', #20263, #499, #16814 ) ;
#23104=CARTESIAN_POINT ( 'NONE',  ( -3.999999999708153453, 38.99999999900385461, -29.00000000000000355 ) ) ;
#23106=DIRECTION ( 'NONE',  ( -1.000000000000000000, 0.000000000000000000, 0.000000000000000000 ) ) ;
#23129=ORIENTED_EDGE ( 'NONE', *, *, #17401, .F. ) ;
#23140=CARTESIAN_POINT ( 'NONE',  ( -3.999999999708139686, 13.32455531934060744, -15.99999999999999289 ) ) ;
#23154=ORIENTED_EDGE ( 'NONE', *, *, #15102, .F. ) ;
#23162=DIRECTION ( 'NONE',  ( 0.000000000000000000, 0.000000000000000000, -1.000000000000000000 ) ) ;
#23168=DIRECTION ( 'NONE',  ( 0.000000000000000000, 0.000000000000000000, -1.000000000000000000 ) ) ;
#23185=VECTOR ( 'NONE', #5946, 1000.000000000000000 ) ;
#23189=DIRECTION ( 'NONE',  ( 0.000000000000000000, -0.000000000000000000, 1.000000000000000000 ) ) ;
#23208=CIRCLE ( 'NONE', #20948, 6.999999999999999112 ) ;
#23209=ORIENTED_EDGE ( 'NONE', *, *, #16619, .T. ) ;
#23218=DIRECTION ( 'NONE',  ( -0.000000000000000000, -0.000000000000000000, -1.000000000000000000 ) ) ;
#23229=CIRCLE ( 'NONE', #1412, 6.500000000000005329 ) ;
#23242=ORIENTED_EDGE ( 'NONE', *, *, #16873, .T. ) ;
#23244=EDGE_LOOP ( 'NONE', ( #4948, #14387, #17844, #21593 ) ) ;
#23254=DIRECTION ( 'NONE',  ( 0.000000000000000000, 0.000000000000000000, -1.000000000000000000 ) ) ;
#23256=COLOUR_RGB ( '', 0.09019608, 0.27058824, 0.51372549) ;
#23259=CARTESIAN_POINT ( 'NONE',  ( -6.683546854663853232, 13.99327871316343952, -17.64411577037000356 ) ) ;
#23260=FACE_OUTER_BOUND ( 'NONE', #4260, .T. ) ;
ENDSEC;
END-ISO-10303-21;
